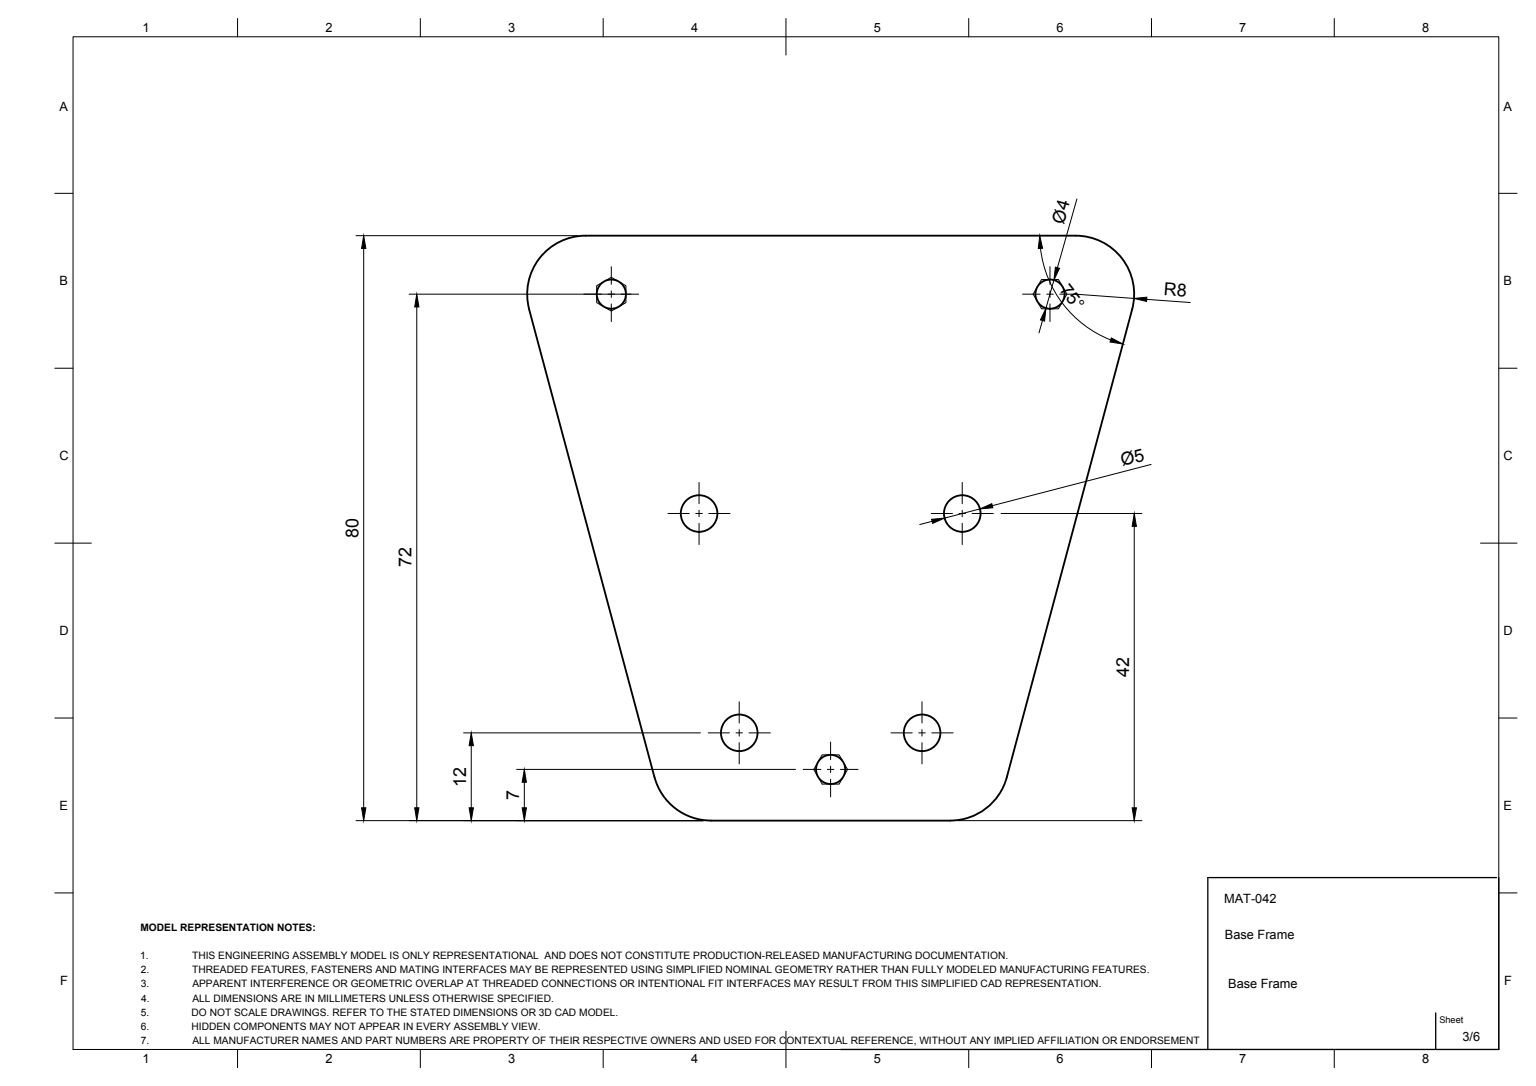
ISO-10303-21;
HEADER;
/* Generated by software containing ST-Developer
 * from STEP Tools, Inc. (www.steptools.com) 
 */

FILE_DESCRIPTION(
/* description */ ('STEP AP214'),
/* implementation_level */ '2;1');

FILE_NAME(
/* name */ 'Base Frame.step',
/* time_stamp */ '2026-11-14T22:03:06-08:00',
/* author */ (''),
/* organization */ (''),
/* preprocessor_version */ 'ST-DEVELOPER v20.2',
/* originating_system */ 'Autodesk Translation Framework v15.17.0.0',
/* authorisation */ '');

FILE_SCHEMA (('AUTOMOTIVE_DESIGN { 1 0 10303 214 3 1 1 }'));
ENDSEC;

DATA;
#10=MECHANICAL_DESIGN_GEOMETRIC_PRESENTATION_REPRESENTATION('',(#303,#304,#305,#306,#307),#12966);
#287=SHAPE_REPRESENTATION_RELATIONSHIP('SRR','None',#13025,#295);
#295=ADVANCED_BREP_SHAPE_REPRESENTATION('',(#315,#316,#317,#318,#319),#12958);
#303=STYLED_ITEM('',(#13074),#315);
#304=STYLED_ITEM('',(#13074),#316);
#305=STYLED_ITEM('',(#13074),#317);
#306=STYLED_ITEM('',(#13074),#318);
#307=STYLED_ITEM('',(#13074),#319);
#315=MANIFOLD_SOLID_BREP('Body1',#5578);
#316=MANIFOLD_SOLID_BREP('Body2',#5579);
#317=MANIFOLD_SOLID_BREP('Body3',#5580);
#318=MANIFOLD_SOLID_BREP('Body4',#5581);
#319=MANIFOLD_SOLID_BREP('Body5',#5582);
#327=FACE_BOUND('',#877,.T.);
#328=FACE_BOUND('',#878,.T.);
#329=FACE_BOUND('',#879,.T.);
#330=FACE_BOUND('',#880,.T.);
#331=FACE_BOUND('',#881,.T.);
#332=FACE_BOUND('',#882,.T.);
#333=FACE_BOUND('',#883,.T.);
#334=FACE_BOUND('',#885,.T.);
#335=FACE_BOUND('',#886,.T.);
#336=FACE_BOUND('',#887,.T.);
#337=FACE_BOUND('',#888,.T.);
#338=FACE_BOUND('',#889,.T.);
#339=FACE_BOUND('',#890,.T.);
#340=FACE_BOUND('',#891,.T.);
#341=FACE_BOUND('',#908,.T.);
#342=FACE_BOUND('',#909,.T.);
#343=FACE_BOUND('',#910,.T.);
#344=FACE_BOUND('',#911,.T.);
#345=FACE_BOUND('',#912,.T.);
#346=FACE_BOUND('',#913,.T.);
#347=FACE_BOUND('',#914,.T.);
#348=FACE_BOUND('',#916,.T.);
#349=FACE_BOUND('',#917,.T.);
#350=FACE_BOUND('',#918,.T.);
#351=FACE_BOUND('',#919,.T.);
#352=FACE_BOUND('',#920,.T.);
#353=FACE_BOUND('',#921,.T.);
#354=FACE_BOUND('',#922,.T.);
#389=PLANE('',#5705);
#390=PLANE('',#5709);
#391=PLANE('',#5713);
#392=PLANE('',#5717);
#393=PLANE('',#5718);
#394=PLANE('',#5719);
#395=PLANE('',#5744);
#396=PLANE('',#5748);
#397=PLANE('',#5752);
#398=PLANE('',#5756);
#399=PLANE('',#5757);
#400=PLANE('',#5758);
#401=PLANE('',#5759);
#402=PLANE('',#5760);
#403=PLANE('',#5761);
#404=PLANE('',#5762);
#405=PLANE('',#5763);
#406=PLANE('',#5764);
#407=PLANE('',#5765);
#408=PLANE('',#5766);
#409=PLANE('',#5767);
#410=PLANE('',#5768);
#411=PLANE('',#5769);
#412=PLANE('',#5770);
#413=PLANE('',#5771);
#414=PLANE('',#5772);
#415=PLANE('',#5773);
#416=PLANE('',#5774);
#417=PLANE('',#5775);
#418=PLANE('',#5776);
#419=PLANE('',#5777);
#420=PLANE('',#5778);
#421=PLANE('',#5779);
#422=PLANE('',#5780);
#423=PLANE('',#5781);
#424=PLANE('',#5782);
#550=FACE_OUTER_BOUND('',#861,.T.);
#551=FACE_OUTER_BOUND('',#862,.T.);
#552=FACE_OUTER_BOUND('',#863,.T.);
#553=FACE_OUTER_BOUND('',#864,.T.);
#554=FACE_OUTER_BOUND('',#865,.T.);
#555=FACE_OUTER_BOUND('',#866,.T.);
#556=FACE_OUTER_BOUND('',#867,.T.);
#557=FACE_OUTER_BOUND('',#868,.T.);
#558=FACE_OUTER_BOUND('',#869,.T.);
#559=FACE_OUTER_BOUND('',#870,.T.);
#560=FACE_OUTER_BOUND('',#871,.T.);
#561=FACE_OUTER_BOUND('',#872,.T.);
#562=FACE_OUTER_BOUND('',#873,.T.);
#563=FACE_OUTER_BOUND('',#874,.T.);
#564=FACE_OUTER_BOUND('',#875,.T.);
#565=FACE_OUTER_BOUND('',#876,.T.);
#566=FACE_OUTER_BOUND('',#884,.T.);
#567=FACE_OUTER_BOUND('',#892,.T.);
#568=FACE_OUTER_BOUND('',#893,.T.);
#569=FACE_OUTER_BOUND('',#894,.T.);
#570=FACE_OUTER_BOUND('',#895,.T.);
#571=FACE_OUTER_BOUND('',#896,.T.);
#572=FACE_OUTER_BOUND('',#897,.T.);
#573=FACE_OUTER_BOUND('',#898,.T.);
#574=FACE_OUTER_BOUND('',#899,.T.);
#575=FACE_OUTER_BOUND('',#900,.T.);
#576=FACE_OUTER_BOUND('',#901,.T.);
#577=FACE_OUTER_BOUND('',#902,.T.);
#578=FACE_OUTER_BOUND('',#903,.T.);
#579=FACE_OUTER_BOUND('',#904,.T.);
#580=FACE_OUTER_BOUND('',#905,.T.);
#581=FACE_OUTER_BOUND('',#906,.T.);
#582=FACE_OUTER_BOUND('',#907,.T.);
#583=FACE_OUTER_BOUND('',#915,.T.);
#584=FACE_OUTER_BOUND('',#923,.T.);
#585=FACE_OUTER_BOUND('',#924,.T.);
#586=FACE_OUTER_BOUND('',#925,.T.);
#587=FACE_OUTER_BOUND('',#926,.T.);
#588=FACE_OUTER_BOUND('',#927,.T.);
#589=FACE_OUTER_BOUND('',#928,.T.);
#590=FACE_OUTER_BOUND('',#929,.T.);
#591=FACE_OUTER_BOUND('',#930,.T.);
#592=FACE_OUTER_BOUND('',#931,.T.);
#593=FACE_OUTER_BOUND('',#932,.T.);
#594=FACE_OUTER_BOUND('',#933,.T.);
#595=FACE_OUTER_BOUND('',#934,.T.);
#596=FACE_OUTER_BOUND('',#935,.T.);
#597=FACE_OUTER_BOUND('',#936,.T.);
#598=FACE_OUTER_BOUND('',#937,.T.);
#599=FACE_OUTER_BOUND('',#938,.T.);
#600=FACE_OUTER_BOUND('',#939,.T.);
#601=FACE_OUTER_BOUND('',#940,.T.);
#602=FACE_OUTER_BOUND('',#941,.T.);
#603=FACE_OUTER_BOUND('',#942,.T.);
#604=FACE_OUTER_BOUND('',#943,.T.);
#605=FACE_OUTER_BOUND('',#944,.T.);
#606=FACE_OUTER_BOUND('',#945,.T.);
#607=FACE_OUTER_BOUND('',#946,.T.);
#861=EDGE_LOOP('',(#3643,#3644,#3645,#3646));
#862=EDGE_LOOP('',(#3647,#3648,#3649,#3650));
#863=EDGE_LOOP('',(#3651,#3652,#3653,#3654));
#864=EDGE_LOOP('',(#3655,#3656,#3657,#3658));
#865=EDGE_LOOP('',(#3659,#3660,#3661,#3662));
#866=EDGE_LOOP('',(#3663,#3664,#3665,#3666));
#867=EDGE_LOOP('',(#3667,#3668,#3669,#3670));
#868=EDGE_LOOP('',(#3671,#3672,#3673,#3674));
#869=EDGE_LOOP('',(#3675,#3676,#3677,#3678));
#870=EDGE_LOOP('',(#3679,#3680,#3681,#3682));
#871=EDGE_LOOP('',(#3683,#3684,#3685,#3686));
#872=EDGE_LOOP('',(#3687,#3688,#3689,#3690));
#873=EDGE_LOOP('',(#3691,#3692,#3693,#3694));
#874=EDGE_LOOP('',(#3695,#3696,#3697,#3698));
#875=EDGE_LOOP('',(#3699,#3700,#3701,#3702));
#876=EDGE_LOOP('',(#3703,#3704,#3705,#3706,#3707,#3708,#3709,#3710));
#877=EDGE_LOOP('',(#3711));
#878=EDGE_LOOP('',(#3712));
#879=EDGE_LOOP('',(#3713));
#880=EDGE_LOOP('',(#3714));
#881=EDGE_LOOP('',(#3715));
#882=EDGE_LOOP('',(#3716));
#883=EDGE_LOOP('',(#3717));
#884=EDGE_LOOP('',(#3718,#3719,#3720,#3721,#3722,#3723,#3724,#3725));
#885=EDGE_LOOP('',(#3726));
#886=EDGE_LOOP('',(#3727));
#887=EDGE_LOOP('',(#3728));
#888=EDGE_LOOP('',(#3729));
#889=EDGE_LOOP('',(#3730));
#890=EDGE_LOOP('',(#3731));
#891=EDGE_LOOP('',(#3732));
#892=EDGE_LOOP('',(#3733,#3734,#3735,#3736));
#893=EDGE_LOOP('',(#3737,#3738,#3739,#3740));
#894=EDGE_LOOP('',(#3741,#3742,#3743,#3744));
#895=EDGE_LOOP('',(#3745,#3746,#3747,#3748));
#896=EDGE_LOOP('',(#3749,#3750,#3751,#3752));
#897=EDGE_LOOP('',(#3753,#3754,#3755,#3756));
#898=EDGE_LOOP('',(#3757,#3758,#3759,#3760));
#899=EDGE_LOOP('',(#3761,#3762,#3763,#3764));
#900=EDGE_LOOP('',(#3765,#3766,#3767,#3768));
#901=EDGE_LOOP('',(#3769,#3770,#3771,#3772));
#902=EDGE_LOOP('',(#3773,#3774,#3775,#3776));
#903=EDGE_LOOP('',(#3777,#3778,#3779,#3780));
#904=EDGE_LOOP('',(#3781,#3782,#3783,#3784));
#905=EDGE_LOOP('',(#3785,#3786,#3787,#3788));
#906=EDGE_LOOP('',(#3789,#3790,#3791,#3792));
#907=EDGE_LOOP('',(#3793,#3794,#3795,#3796,#3797,#3798,#3799,#3800));
#908=EDGE_LOOP('',(#3801));
#909=EDGE_LOOP('',(#3802));
#910=EDGE_LOOP('',(#3803));
#911=EDGE_LOOP('',(#3804));
#912=EDGE_LOOP('',(#3805));
#913=EDGE_LOOP('',(#3806));
#914=EDGE_LOOP('',(#3807));
#915=EDGE_LOOP('',(#3808,#3809,#3810,#3811,#3812,#3813,#3814,#3815));
#916=EDGE_LOOP('',(#3816));
#917=EDGE_LOOP('',(#3817));
#918=EDGE_LOOP('',(#3818));
#919=EDGE_LOOP('',(#3819));
#920=EDGE_LOOP('',(#3820));
#921=EDGE_LOOP('',(#3821));
#922=EDGE_LOOP('',(#3822));
#923=EDGE_LOOP('',(#3823,#3824,#3825,#3826));
#924=EDGE_LOOP('',(#3827,#3828,#3829,#3830));
#925=EDGE_LOOP('',(#3831,#3832,#3833,#3834));
#926=EDGE_LOOP('',(#3835,#3836,#3837,#3838));
#927=EDGE_LOOP('',(#3839,#3840,#3841,#3842));
#928=EDGE_LOOP('',(#3843,#3844,#3845,#3846));
#929=EDGE_LOOP('',(#3847,#3848,#3849,#3850,#3851,#3852));
#930=EDGE_LOOP('',(#3853,#3854,#3855,#3856,#3857,#3858));
#931=EDGE_LOOP('',(#3859,#3860,#3861,#3862));
#932=EDGE_LOOP('',(#3863,#3864,#3865,#3866));
#933=EDGE_LOOP('',(#3867,#3868,#3869,#3870));
#934=EDGE_LOOP('',(#3871,#3872,#3873,#3874));
#935=EDGE_LOOP('',(#3875,#3876,#3877,#3878));
#936=EDGE_LOOP('',(#3879,#3880,#3881,#3882));
#937=EDGE_LOOP('',(#3883,#3884,#3885,#3886,#3887,#3888));
#938=EDGE_LOOP('',(#3889,#3890,#3891,#3892,#3893,#3894));
#939=EDGE_LOOP('',(#3895,#3896,#3897,#3898));
#940=EDGE_LOOP('',(#3899,#3900,#3901,#3902));
#941=EDGE_LOOP('',(#3903,#3904,#3905,#3906));
#942=EDGE_LOOP('',(#3907,#3908,#3909,#3910));
#943=EDGE_LOOP('',(#3911,#3912,#3913,#3914));
#944=EDGE_LOOP('',(#3915,#3916,#3917,#3918));
#945=EDGE_LOOP('',(#3919,#3920,#3921,#3922,#3923,#3924));
#946=EDGE_LOOP('',(#3925,#3926,#3927,#3928,#3929,#3930));
#1234=LINE('',#7771,#1691);
#1235=LINE('',#7777,#1692);
#1236=LINE('',#7783,#1693);
#1237=LINE('',#7789,#1694);
#1238=LINE('',#7795,#1695);
#1239=LINE('',#7801,#1696);
#1240=LINE('',#7807,#1697);
#1241=LINE('',#7814,#1698);
#1242=LINE('',#7817,#1699);
#1243=LINE('',#7820,#1700);
#1244=LINE('',#7822,#1701);
#1245=LINE('',#7823,#1702);
#1246=LINE('',#7828,#1703);
#1247=LINE('',#7832,#1704);
#1248=LINE('',#7834,#1705);
#1249=LINE('',#7835,#1706);
#1250=LINE('',#7840,#1707);
#1251=LINE('',#7844,#1708);
#1252=LINE('',#7846,#1709);
#1253=LINE('',#7847,#1710);
#1254=LINE('',#7852,#1711);
#1255=LINE('',#7855,#1712);
#1256=LINE('',#7856,#1713);
#1257=LINE('',#7863,#1714);
#1258=LINE('',#7869,#1715);
#1259=LINE('',#7875,#1716);
#1260=LINE('',#7881,#1717);
#1261=LINE('',#7888,#1718);
#1262=LINE('',#7891,#1719);
#1263=LINE('',#7896,#1720);
#1264=LINE('',#7902,#1721);
#1265=LINE('',#7908,#1722);
#1266=LINE('',#7912,#1723);
#1267=LINE('',#7914,#1724);
#1268=LINE('',#7915,#1725);
#1269=LINE('',#7920,#1726);
#1270=LINE('',#7924,#1727);
#1271=LINE('',#7926,#1728);
#1272=LINE('',#7927,#1729);
#1273=LINE('',#7932,#1730);
#1274=LINE('',#7936,#1731);
#1275=LINE('',#7938,#1732);
#1276=LINE('',#7939,#1733);
#1277=LINE('',#7944,#1734);
#1278=LINE('',#7947,#1735);
#1279=LINE('',#7948,#1736);
#1280=LINE('',#7954,#1737);
#1281=LINE('',#7956,#1738);
#1282=LINE('',#7958,#1739);
#1283=LINE('',#7959,#1740);
#1284=LINE('',#7962,#1741);
#1285=LINE('',#7964,#1742);
#1286=LINE('',#7965,#1743);
#1287=LINE('',#7968,#1744);
#1288=LINE('',#7970,#1745);
#1289=LINE('',#7971,#1746);
#1290=LINE('',#7974,#1747);
#1291=LINE('',#7976,#1748);
#1292=LINE('',#7977,#1749);
#1293=LINE('',#7980,#1750);
#1294=LINE('',#7982,#1751);
#1295=LINE('',#7983,#1752);
#1296=LINE('',#7985,#1753);
#1297=LINE('',#7986,#1754);
#1298=LINE('',#7992,#1755);
#1299=LINE('',#7994,#1756);
#1300=LINE('',#7996,#1757);
#1301=LINE('',#7997,#1758);
#1302=LINE('',#8000,#1759);
#1303=LINE('',#8002,#1760);
#1304=LINE('',#8003,#1761);
#1305=LINE('',#8006,#1762);
#1306=LINE('',#8008,#1763);
#1307=LINE('',#8009,#1764);
#1308=LINE('',#8012,#1765);
#1309=LINE('',#8014,#1766);
#1310=LINE('',#8015,#1767);
#1311=LINE('',#8018,#1768);
#1312=LINE('',#8020,#1769);
#1313=LINE('',#8021,#1770);
#1314=LINE('',#8023,#1771);
#1315=LINE('',#8024,#1772);
#1316=LINE('',#8030,#1773);
#1317=LINE('',#8032,#1774);
#1318=LINE('',#8034,#1775);
#1319=LINE('',#8035,#1776);
#1320=LINE('',#8038,#1777);
#1321=LINE('',#8040,#1778);
#1322=LINE('',#8041,#1779);
#1323=LINE('',#8044,#1780);
#1324=LINE('',#8046,#1781);
#1325=LINE('',#8047,#1782);
#1326=LINE('',#8050,#1783);
#1327=LINE('',#8052,#1784);
#1328=LINE('',#8053,#1785);
#1329=LINE('',#8056,#1786);
#1330=LINE('',#8058,#1787);
#1331=LINE('',#8059,#1788);
#1332=LINE('',#8061,#1789);
#1333=LINE('',#8062,#1790);
#1691=VECTOR('',#6230,1.99999999999998);
#1692=VECTOR('',#6237,1.99999999999998);
#1693=VECTOR('',#6244,2.);
#1694=VECTOR('',#6251,2.5);
#1695=VECTOR('',#6258,2.5);
#1696=VECTOR('',#6265,2.5);
#1697=VECTOR('',#6272,2.5);
#1698=VECTOR('',#6279,1000.);
#1699=VECTOR('',#6282,1000.);
#1700=VECTOR('',#6285,1000.);
#1701=VECTOR('',#6286,1000.);
#1702=VECTOR('',#6287,1000.);
#1703=VECTOR('',#6292,1000.);
#1704=VECTOR('',#6297,1000.);
#1705=VECTOR('',#6298,1000.);
#1706=VECTOR('',#6299,1000.);
#1707=VECTOR('',#6304,1000.);
#1708=VECTOR('',#6309,1000.);
#1709=VECTOR('',#6310,1000.);
#1710=VECTOR('',#6311,1000.);
#1711=VECTOR('',#6316,1000.);
#1712=VECTOR('',#6321,1000.);
#1713=VECTOR('',#6322,1000.);
#1714=VECTOR('',#6331,1.99999999999998);
#1715=VECTOR('',#6338,1.99999999999998);
#1716=VECTOR('',#6345,2.5);
#1717=VECTOR('',#6352,2.5);
#1718=VECTOR('',#6359,1000.);
#1719=VECTOR('',#6362,1000.);
#1720=VECTOR('',#6367,2.5);
#1721=VECTOR('',#6374,2.5);
#1722=VECTOR('',#6381,2.);
#1723=VECTOR('',#6386,1000.);
#1724=VECTOR('',#6387,1000.);
#1725=VECTOR('',#6388,1000.);
#1726=VECTOR('',#6393,1000.);
#1727=VECTOR('',#6398,1000.);
#1728=VECTOR('',#6399,1000.);
#1729=VECTOR('',#6400,1000.);
#1730=VECTOR('',#6405,1000.);
#1731=VECTOR('',#6410,1000.);
#1732=VECTOR('',#6411,1000.);
#1733=VECTOR('',#6412,1000.);
#1734=VECTOR('',#6417,1000.);
#1735=VECTOR('',#6422,1000.);
#1736=VECTOR('',#6423,1000.);
#1737=VECTOR('',#6430,1000.);
#1738=VECTOR('',#6431,1000.);
#1739=VECTOR('',#6432,1000.);
#1740=VECTOR('',#6433,1000.);
#1741=VECTOR('',#6436,1000.);
#1742=VECTOR('',#6437,1000.);
#1743=VECTOR('',#6438,1000.);
#1744=VECTOR('',#6441,1000.);
#1745=VECTOR('',#6442,1000.);
#1746=VECTOR('',#6443,1000.);
#1747=VECTOR('',#6446,1000.);
#1748=VECTOR('',#6447,1000.);
#1749=VECTOR('',#6448,1000.);
#1750=VECTOR('',#6451,1000.);
#1751=VECTOR('',#6452,1000.);
#1752=VECTOR('',#6453,1000.);
#1753=VECTOR('',#6456,1000.);
#1754=VECTOR('',#6457,1000.);
#1755=VECTOR('',#6464,1000.);
#1756=VECTOR('',#6465,1000.);
#1757=VECTOR('',#6466,1000.);
#1758=VECTOR('',#6467,1000.);
#1759=VECTOR('',#6470,1000.);
#1760=VECTOR('',#6471,1000.);
#1761=VECTOR('',#6472,1000.);
#1762=VECTOR('',#6475,1000.);
#1763=VECTOR('',#6476,1000.);
#1764=VECTOR('',#6477,1000.);
#1765=VECTOR('',#6480,1000.);
#1766=VECTOR('',#6481,1000.);
#1767=VECTOR('',#6482,1000.);
#1768=VECTOR('',#6485,1000.);
#1769=VECTOR('',#6486,1000.);
#1770=VECTOR('',#6487,1000.);
#1771=VECTOR('',#6490,1000.);
#1772=VECTOR('',#6491,1000.);
#1773=VECTOR('',#6498,1000.);
#1774=VECTOR('',#6499,1000.);
#1775=VECTOR('',#6500,1000.);
#1776=VECTOR('',#6501,1000.);
#1777=VECTOR('',#6504,1000.);
#1778=VECTOR('',#6505,1000.);
#1779=VECTOR('',#6506,1000.);
#1780=VECTOR('',#6509,1000.);
#1781=VECTOR('',#6510,1000.);
#1782=VECTOR('',#6511,1000.);
#1783=VECTOR('',#6514,1000.);
#1784=VECTOR('',#6515,1000.);
#1785=VECTOR('',#6516,1000.);
#1786=VECTOR('',#6519,1000.);
#1787=VECTOR('',#6520,1000.);
#1788=VECTOR('',#6521,1000.);
#1789=VECTOR('',#6524,1000.);
#1790=VECTOR('',#6525,1000.);
#2148=CIRCLE('',#5682,1.99999999999998);
#2149=CIRCLE('',#5683,1.99999999999997);
#2150=CIRCLE('',#5685,1.99999999999998);
#2151=CIRCLE('',#5686,1.99999999999997);
#2152=CIRCLE('',#5688,2.);
#2153=CIRCLE('',#5689,2.);
#2154=CIRCLE('',#5691,2.5);
#2155=CIRCLE('',#5692,2.5);
#2156=CIRCLE('',#5694,2.5);
#2157=CIRCLE('',#5695,2.5);
#2158=CIRCLE('',#5697,2.5);
#2159=CIRCLE('',#5698,2.5);
#2160=CIRCLE('',#5700,2.5);
#2161=CIRCLE('',#5701,2.5);
#2162=CIRCLE('',#5703,8.);
#2163=CIRCLE('',#5704,8.00000000000001);
#2164=CIRCLE('',#5707,8.);
#2165=CIRCLE('',#5708,8.);
#2166=CIRCLE('',#5711,8.);
#2167=CIRCLE('',#5712,8.);
#2168=CIRCLE('',#5715,8.00000000000001);
#2169=CIRCLE('',#5716,8.00000000000001);
#2170=CIRCLE('',#5721,1.99999999999998);
#2171=CIRCLE('',#5722,1.99999999999998);
#2172=CIRCLE('',#5724,1.99999999999998);
#2173=CIRCLE('',#5725,1.99999999999998);
#2174=CIRCLE('',#5727,2.5);
#2175=CIRCLE('',#5728,2.5);
#2176=CIRCLE('',#5730,2.5);
#2177=CIRCLE('',#5731,2.5);
#2178=CIRCLE('',#5733,8.00000000000001);
#2179=CIRCLE('',#5734,8.);
#2180=CIRCLE('',#5736,2.5);
#2181=CIRCLE('',#5737,2.5);
#2182=CIRCLE('',#5739,2.5);
#2183=CIRCLE('',#5740,2.5);
#2184=CIRCLE('',#5742,2.);
#2185=CIRCLE('',#5743,2.);
#2186=CIRCLE('',#5746,8.);
#2187=CIRCLE('',#5747,8.00000000000001);
#2188=CIRCLE('',#5750,8.);
#2189=CIRCLE('',#5751,8.);
#2190=CIRCLE('',#5754,8.);
#2191=CIRCLE('',#5755,8.);
#2376=VERTEX_POINT('',#7768);
#2377=VERTEX_POINT('',#7770);
#2378=VERTEX_POINT('',#7774);
#2379=VERTEX_POINT('',#7776);
#2380=VERTEX_POINT('',#7780);
#2381=VERTEX_POINT('',#7782);
#2382=VERTEX_POINT('',#7786);
#2383=VERTEX_POINT('',#7788);
#2384=VERTEX_POINT('',#7792);
#2385=VERTEX_POINT('',#7794);
#2386=VERTEX_POINT('',#7798);
#2387=VERTEX_POINT('',#7800);
#2388=VERTEX_POINT('',#7804);
#2389=VERTEX_POINT('',#7806);
#2390=VERTEX_POINT('',#7810);
#2391=VERTEX_POINT('',#7811);
#2392=VERTEX_POINT('',#7813);
#2393=VERTEX_POINT('',#7815);
#2394=VERTEX_POINT('',#7819);
#2395=VERTEX_POINT('',#7821);
#2396=VERTEX_POINT('',#7825);
#2397=VERTEX_POINT('',#7827);
#2398=VERTEX_POINT('',#7831);
#2399=VERTEX_POINT('',#7833);
#2400=VERTEX_POINT('',#7837);
#2401=VERTEX_POINT('',#7839);
#2402=VERTEX_POINT('',#7843);
#2403=VERTEX_POINT('',#7845);
#2404=VERTEX_POINT('',#7849);
#2405=VERTEX_POINT('',#7851);
#2406=VERTEX_POINT('',#7860);
#2407=VERTEX_POINT('',#7862);
#2408=VERTEX_POINT('',#7866);
#2409=VERTEX_POINT('',#7868);
#2410=VERTEX_POINT('',#7872);
#2411=VERTEX_POINT('',#7874);
#2412=VERTEX_POINT('',#7878);
#2413=VERTEX_POINT('',#7880);
#2414=VERTEX_POINT('',#7884);
#2415=VERTEX_POINT('',#7885);
#2416=VERTEX_POINT('',#7887);
#2417=VERTEX_POINT('',#7889);
#2418=VERTEX_POINT('',#7893);
#2419=VERTEX_POINT('',#7895);
#2420=VERTEX_POINT('',#7899);
#2421=VERTEX_POINT('',#7901);
#2422=VERTEX_POINT('',#7905);
#2423=VERTEX_POINT('',#7907);
#2424=VERTEX_POINT('',#7911);
#2425=VERTEX_POINT('',#7913);
#2426=VERTEX_POINT('',#7917);
#2427=VERTEX_POINT('',#7919);
#2428=VERTEX_POINT('',#7923);
#2429=VERTEX_POINT('',#7925);
#2430=VERTEX_POINT('',#7929);
#2431=VERTEX_POINT('',#7931);
#2432=VERTEX_POINT('',#7935);
#2433=VERTEX_POINT('',#7937);
#2434=VERTEX_POINT('',#7941);
#2435=VERTEX_POINT('',#7943);
#2436=VERTEX_POINT('',#7952);
#2437=VERTEX_POINT('',#7953);
#2438=VERTEX_POINT('',#7955);
#2439=VERTEX_POINT('',#7957);
#2440=VERTEX_POINT('',#7961);
#2441=VERTEX_POINT('',#7963);
#2442=VERTEX_POINT('',#7967);
#2443=VERTEX_POINT('',#7969);
#2444=VERTEX_POINT('',#7973);
#2445=VERTEX_POINT('',#7975);
#2446=VERTEX_POINT('',#7979);
#2447=VERTEX_POINT('',#7981);
#2448=VERTEX_POINT('',#7990);
#2449=VERTEX_POINT('',#7991);
#2450=VERTEX_POINT('',#7993);
#2451=VERTEX_POINT('',#7995);
#2452=VERTEX_POINT('',#7999);
#2453=VERTEX_POINT('',#8001);
#2454=VERTEX_POINT('',#8005);
#2455=VERTEX_POINT('',#8007);
#2456=VERTEX_POINT('',#8011);
#2457=VERTEX_POINT('',#8013);
#2458=VERTEX_POINT('',#8017);
#2459=VERTEX_POINT('',#8019);
#2460=VERTEX_POINT('',#8028);
#2461=VERTEX_POINT('',#8029);
#2462=VERTEX_POINT('',#8031);
#2463=VERTEX_POINT('',#8033);
#2464=VERTEX_POINT('',#8037);
#2465=VERTEX_POINT('',#8039);
#2466=VERTEX_POINT('',#8043);
#2467=VERTEX_POINT('',#8045);
#2468=VERTEX_POINT('',#8049);
#2469=VERTEX_POINT('',#8051);
#2470=VERTEX_POINT('',#8055);
#2471=VERTEX_POINT('',#8057);
#2878=EDGE_CURVE('',#2376,#2376,#2148,.T.);
#2879=EDGE_CURVE('',#2376,#2377,#1234,.T.);
#2880=EDGE_CURVE('',#2377,#2377,#2149,.T.);
#2881=EDGE_CURVE('',#2378,#2378,#2150,.T.);
#2882=EDGE_CURVE('',#2378,#2379,#1235,.T.);
#2883=EDGE_CURVE('',#2379,#2379,#2151,.T.);
#2884=EDGE_CURVE('',#2380,#2380,#2152,.T.);
#2885=EDGE_CURVE('',#2380,#2381,#1236,.T.);
#2886=EDGE_CURVE('',#2381,#2381,#2153,.T.);
#2887=EDGE_CURVE('',#2382,#2382,#2154,.T.);
#2888=EDGE_CURVE('',#2382,#2383,#1237,.T.);
#2889=EDGE_CURVE('',#2383,#2383,#2155,.T.);
#2890=EDGE_CURVE('',#2384,#2384,#2156,.T.);
#2891=EDGE_CURVE('',#2384,#2385,#1238,.T.);
#2892=EDGE_CURVE('',#2385,#2385,#2157,.T.);
#2893=EDGE_CURVE('',#2386,#2386,#2158,.T.);
#2894=EDGE_CURVE('',#2386,#2387,#1239,.T.);
#2895=EDGE_CURVE('',#2387,#2387,#2159,.T.);
#2896=EDGE_CURVE('',#2388,#2388,#2160,.T.);
#2897=EDGE_CURVE('',#2388,#2389,#1240,.T.);
#2898=EDGE_CURVE('',#2389,#2389,#2161,.T.);
#2899=EDGE_CURVE('',#2390,#2391,#2162,.T.);
#2900=EDGE_CURVE('',#2390,#2392,#1241,.T.);
#2901=EDGE_CURVE('',#2392,#2393,#2163,.T.);
#2902=EDGE_CURVE('',#2391,#2393,#1242,.T.);
#2903=EDGE_CURVE('',#2393,#2394,#1243,.T.);
#2904=EDGE_CURVE('',#2395,#2394,#1244,.T.);
#2905=EDGE_CURVE('',#2391,#2395,#1245,.T.);
#2906=EDGE_CURVE('',#2394,#2396,#2164,.T.);
#2907=EDGE_CURVE('',#2397,#2396,#1246,.T.);
#2908=EDGE_CURVE('',#2395,#2397,#2165,.T.);
#2909=EDGE_CURVE('',#2396,#2398,#1247,.T.);
#2910=EDGE_CURVE('',#2399,#2398,#1248,.T.);
#2911=EDGE_CURVE('',#2397,#2399,#1249,.T.);
#2912=EDGE_CURVE('',#2398,#2400,#2166,.T.);
#2913=EDGE_CURVE('',#2401,#2400,#1250,.T.);
#2914=EDGE_CURVE('',#2399,#2401,#2167,.T.);
#2915=EDGE_CURVE('',#2400,#2402,#1251,.T.);
#2916=EDGE_CURVE('',#2403,#2402,#1252,.T.);
#2917=EDGE_CURVE('',#2401,#2403,#1253,.T.);
#2918=EDGE_CURVE('',#2402,#2404,#2168,.T.);
#2919=EDGE_CURVE('',#2405,#2404,#1254,.T.);
#2920=EDGE_CURVE('',#2403,#2405,#2169,.T.);
#2921=EDGE_CURVE('',#2392,#2404,#1255,.T.);
#2922=EDGE_CURVE('',#2405,#2390,#1256,.T.);
#2923=EDGE_CURVE('',#2406,#2406,#2170,.T.);
#2924=EDGE_CURVE('',#2406,#2407,#1257,.T.);
#2925=EDGE_CURVE('',#2407,#2407,#2171,.T.);
#2926=EDGE_CURVE('',#2408,#2408,#2172,.T.);
#2927=EDGE_CURVE('',#2408,#2409,#1258,.T.);
#2928=EDGE_CURVE('',#2409,#2409,#2173,.T.);
#2929=EDGE_CURVE('',#2410,#2410,#2174,.T.);
#2930=EDGE_CURVE('',#2410,#2411,#1259,.T.);
#2931=EDGE_CURVE('',#2411,#2411,#2175,.T.);
#2932=EDGE_CURVE('',#2412,#2412,#2176,.T.);
#2933=EDGE_CURVE('',#2412,#2413,#1260,.T.);
#2934=EDGE_CURVE('',#2413,#2413,#2177,.T.);
#2935=EDGE_CURVE('',#2414,#2415,#2178,.T.);
#2936=EDGE_CURVE('',#2415,#2416,#1261,.T.);
#2937=EDGE_CURVE('',#2416,#2417,#2179,.T.);
#2938=EDGE_CURVE('',#2414,#2417,#1262,.T.);
#2939=EDGE_CURVE('',#2418,#2418,#2180,.T.);
#2940=EDGE_CURVE('',#2418,#2419,#1263,.T.);
#2941=EDGE_CURVE('',#2419,#2419,#2181,.T.);
#2942=EDGE_CURVE('',#2420,#2420,#2182,.T.);
#2943=EDGE_CURVE('',#2420,#2421,#1264,.T.);
#2944=EDGE_CURVE('',#2421,#2421,#2183,.T.);
#2945=EDGE_CURVE('',#2422,#2422,#2184,.T.);
#2946=EDGE_CURVE('',#2422,#2423,#1265,.T.);
#2947=EDGE_CURVE('',#2423,#2423,#2185,.T.);
#2948=EDGE_CURVE('',#2415,#2424,#1266,.T.);
#2949=EDGE_CURVE('',#2424,#2425,#1267,.T.);
#2950=EDGE_CURVE('',#2425,#2416,#1268,.T.);
#2951=EDGE_CURVE('',#2424,#2426,#2186,.T.);
#2952=EDGE_CURVE('',#2426,#2427,#1269,.T.);
#2953=EDGE_CURVE('',#2427,#2425,#2187,.T.);
#2954=EDGE_CURVE('',#2426,#2428,#1270,.T.);
#2955=EDGE_CURVE('',#2428,#2429,#1271,.T.);
#2956=EDGE_CURVE('',#2429,#2427,#1272,.T.);
#2957=EDGE_CURVE('',#2428,#2430,#2188,.T.);
#2958=EDGE_CURVE('',#2430,#2431,#1273,.T.);
#2959=EDGE_CURVE('',#2431,#2429,#2189,.T.);
#2960=EDGE_CURVE('',#2432,#2430,#1274,.T.);
#2961=EDGE_CURVE('',#2432,#2433,#1275,.T.);
#2962=EDGE_CURVE('',#2433,#2431,#1276,.T.);
#2963=EDGE_CURVE('',#2432,#2434,#2190,.T.);
#2964=EDGE_CURVE('',#2434,#2435,#1277,.T.);
#2965=EDGE_CURVE('',#2435,#2433,#2191,.T.);
#2966=EDGE_CURVE('',#2434,#2414,#1278,.T.);
#2967=EDGE_CURVE('',#2417,#2435,#1279,.T.);
#2968=EDGE_CURVE('',#2436,#2437,#1280,.T.);
#2969=EDGE_CURVE('',#2438,#2437,#1281,.T.);
#2970=EDGE_CURVE('',#2439,#2438,#1282,.T.);
#2971=EDGE_CURVE('',#2439,#2436,#1283,.T.);
#2972=EDGE_CURVE('',#2437,#2440,#1284,.T.);
#2973=EDGE_CURVE('',#2441,#2440,#1285,.T.);
#2974=EDGE_CURVE('',#2438,#2441,#1286,.T.);
#2975=EDGE_CURVE('',#2440,#2442,#1287,.T.);
#2976=EDGE_CURVE('',#2443,#2442,#1288,.T.);
#2977=EDGE_CURVE('',#2441,#2443,#1289,.T.);
#2978=EDGE_CURVE('',#2442,#2444,#1290,.T.);
#2979=EDGE_CURVE('',#2445,#2444,#1291,.T.);
#2980=EDGE_CURVE('',#2443,#2445,#1292,.T.);
#2981=EDGE_CURVE('',#2444,#2446,#1293,.T.);
#2982=EDGE_CURVE('',#2447,#2446,#1294,.T.);
#2983=EDGE_CURVE('',#2445,#2447,#1295,.T.);
#2984=EDGE_CURVE('',#2446,#2436,#1296,.T.);
#2985=EDGE_CURVE('',#2447,#2439,#1297,.T.);
#2986=EDGE_CURVE('',#2448,#2449,#1298,.T.);
#2987=EDGE_CURVE('',#2450,#2449,#1299,.T.);
#2988=EDGE_CURVE('',#2451,#2450,#1300,.T.);
#2989=EDGE_CURVE('',#2451,#2448,#1301,.T.);
#2990=EDGE_CURVE('',#2449,#2452,#1302,.T.);
#2991=EDGE_CURVE('',#2453,#2452,#1303,.T.);
#2992=EDGE_CURVE('',#2450,#2453,#1304,.T.);
#2993=EDGE_CURVE('',#2452,#2454,#1305,.T.);
#2994=EDGE_CURVE('',#2455,#2454,#1306,.T.);
#2995=EDGE_CURVE('',#2453,#2455,#1307,.T.);
#2996=EDGE_CURVE('',#2454,#2456,#1308,.T.);
#2997=EDGE_CURVE('',#2457,#2456,#1309,.T.);
#2998=EDGE_CURVE('',#2455,#2457,#1310,.T.);
#2999=EDGE_CURVE('',#2456,#2458,#1311,.T.);
#3000=EDGE_CURVE('',#2459,#2458,#1312,.T.);
#3001=EDGE_CURVE('',#2457,#2459,#1313,.T.);
#3002=EDGE_CURVE('',#2458,#2448,#1314,.T.);
#3003=EDGE_CURVE('',#2459,#2451,#1315,.T.);
#3004=EDGE_CURVE('',#2460,#2461,#1316,.T.);
#3005=EDGE_CURVE('',#2462,#2461,#1317,.T.);
#3006=EDGE_CURVE('',#2463,#2462,#1318,.T.);
#3007=EDGE_CURVE('',#2463,#2460,#1319,.T.);
#3008=EDGE_CURVE('',#2461,#2464,#1320,.T.);
#3009=EDGE_CURVE('',#2465,#2464,#1321,.T.);
#3010=EDGE_CURVE('',#2462,#2465,#1322,.T.);
#3011=EDGE_CURVE('',#2464,#2466,#1323,.T.);
#3012=EDGE_CURVE('',#2467,#2466,#1324,.T.);
#3013=EDGE_CURVE('',#2465,#2467,#1325,.T.);
#3014=EDGE_CURVE('',#2466,#2468,#1326,.T.);
#3015=EDGE_CURVE('',#2469,#2468,#1327,.T.);
#3016=EDGE_CURVE('',#2467,#2469,#1328,.T.);
#3017=EDGE_CURVE('',#2468,#2470,#1329,.T.);
#3018=EDGE_CURVE('',#2471,#2470,#1330,.T.);
#3019=EDGE_CURVE('',#2469,#2471,#1331,.T.);
#3020=EDGE_CURVE('',#2470,#2460,#1332,.T.);
#3021=EDGE_CURVE('',#2471,#2463,#1333,.T.);
#3643=ORIENTED_EDGE('',*,*,#2878,.T.);
#3644=ORIENTED_EDGE('',*,*,#2879,.T.);
#3645=ORIENTED_EDGE('',*,*,#2880,.F.);
#3646=ORIENTED_EDGE('',*,*,#2879,.F.);
#3647=ORIENTED_EDGE('',*,*,#2881,.T.);
#3648=ORIENTED_EDGE('',*,*,#2882,.T.);
#3649=ORIENTED_EDGE('',*,*,#2883,.F.);
#3650=ORIENTED_EDGE('',*,*,#2882,.F.);
#3651=ORIENTED_EDGE('',*,*,#2884,.T.);
#3652=ORIENTED_EDGE('',*,*,#2885,.T.);
#3653=ORIENTED_EDGE('',*,*,#2886,.F.);
#3654=ORIENTED_EDGE('',*,*,#2885,.F.);
#3655=ORIENTED_EDGE('',*,*,#2887,.T.);
#3656=ORIENTED_EDGE('',*,*,#2888,.T.);
#3657=ORIENTED_EDGE('',*,*,#2889,.F.);
#3658=ORIENTED_EDGE('',*,*,#2888,.F.);
#3659=ORIENTED_EDGE('',*,*,#2890,.T.);
#3660=ORIENTED_EDGE('',*,*,#2891,.T.);
#3661=ORIENTED_EDGE('',*,*,#2892,.F.);
#3662=ORIENTED_EDGE('',*,*,#2891,.F.);
#3663=ORIENTED_EDGE('',*,*,#2893,.T.);
#3664=ORIENTED_EDGE('',*,*,#2894,.T.);
#3665=ORIENTED_EDGE('',*,*,#2895,.F.);
#3666=ORIENTED_EDGE('',*,*,#2894,.F.);
#3667=ORIENTED_EDGE('',*,*,#2896,.T.);
#3668=ORIENTED_EDGE('',*,*,#2897,.T.);
#3669=ORIENTED_EDGE('',*,*,#2898,.F.);
#3670=ORIENTED_EDGE('',*,*,#2897,.F.);
#3671=ORIENTED_EDGE('',*,*,#2899,.F.);
#3672=ORIENTED_EDGE('',*,*,#2900,.T.);
#3673=ORIENTED_EDGE('',*,*,#2901,.T.);
#3674=ORIENTED_EDGE('',*,*,#2902,.F.);
#3675=ORIENTED_EDGE('',*,*,#2902,.T.);
#3676=ORIENTED_EDGE('',*,*,#2903,.T.);
#3677=ORIENTED_EDGE('',*,*,#2904,.F.);
#3678=ORIENTED_EDGE('',*,*,#2905,.F.);
#3679=ORIENTED_EDGE('',*,*,#2904,.T.);
#3680=ORIENTED_EDGE('',*,*,#2906,.T.);
#3681=ORIENTED_EDGE('',*,*,#2907,.F.);
#3682=ORIENTED_EDGE('',*,*,#2908,.F.);
#3683=ORIENTED_EDGE('',*,*,#2907,.T.);
#3684=ORIENTED_EDGE('',*,*,#2909,.T.);
#3685=ORIENTED_EDGE('',*,*,#2910,.F.);
#3686=ORIENTED_EDGE('',*,*,#2911,.F.);
#3687=ORIENTED_EDGE('',*,*,#2910,.T.);
#3688=ORIENTED_EDGE('',*,*,#2912,.T.);
#3689=ORIENTED_EDGE('',*,*,#2913,.F.);
#3690=ORIENTED_EDGE('',*,*,#2914,.F.);
#3691=ORIENTED_EDGE('',*,*,#2913,.T.);
#3692=ORIENTED_EDGE('',*,*,#2915,.T.);
#3693=ORIENTED_EDGE('',*,*,#2916,.F.);
#3694=ORIENTED_EDGE('',*,*,#2917,.F.);
#3695=ORIENTED_EDGE('',*,*,#2916,.T.);
#3696=ORIENTED_EDGE('',*,*,#2918,.T.);
#3697=ORIENTED_EDGE('',*,*,#2919,.F.);
#3698=ORIENTED_EDGE('',*,*,#2920,.F.);
#3699=ORIENTED_EDGE('',*,*,#2919,.T.);
#3700=ORIENTED_EDGE('',*,*,#2921,.F.);
#3701=ORIENTED_EDGE('',*,*,#2900,.F.);
#3702=ORIENTED_EDGE('',*,*,#2922,.F.);
#3703=ORIENTED_EDGE('',*,*,#2899,.T.);
#3704=ORIENTED_EDGE('',*,*,#2905,.T.);
#3705=ORIENTED_EDGE('',*,*,#2908,.T.);
#3706=ORIENTED_EDGE('',*,*,#2911,.T.);
#3707=ORIENTED_EDGE('',*,*,#2914,.T.);
#3708=ORIENTED_EDGE('',*,*,#2917,.T.);
#3709=ORIENTED_EDGE('',*,*,#2920,.T.);
#3710=ORIENTED_EDGE('',*,*,#2922,.T.);
#3711=ORIENTED_EDGE('',*,*,#2896,.F.);
#3712=ORIENTED_EDGE('',*,*,#2890,.F.);
#3713=ORIENTED_EDGE('',*,*,#2884,.F.);
#3714=ORIENTED_EDGE('',*,*,#2878,.F.);
#3715=ORIENTED_EDGE('',*,*,#2881,.F.);
#3716=ORIENTED_EDGE('',*,*,#2887,.F.);
#3717=ORIENTED_EDGE('',*,*,#2893,.F.);
#3718=ORIENTED_EDGE('',*,*,#2921,.T.);
#3719=ORIENTED_EDGE('',*,*,#2918,.F.);
#3720=ORIENTED_EDGE('',*,*,#2915,.F.);
#3721=ORIENTED_EDGE('',*,*,#2912,.F.);
#3722=ORIENTED_EDGE('',*,*,#2909,.F.);
#3723=ORIENTED_EDGE('',*,*,#2906,.F.);
#3724=ORIENTED_EDGE('',*,*,#2903,.F.);
#3725=ORIENTED_EDGE('',*,*,#2901,.F.);
#3726=ORIENTED_EDGE('',*,*,#2898,.T.);
#3727=ORIENTED_EDGE('',*,*,#2895,.T.);
#3728=ORIENTED_EDGE('',*,*,#2892,.T.);
#3729=ORIENTED_EDGE('',*,*,#2889,.T.);
#3730=ORIENTED_EDGE('',*,*,#2886,.T.);
#3731=ORIENTED_EDGE('',*,*,#2883,.T.);
#3732=ORIENTED_EDGE('',*,*,#2880,.T.);
#3733=ORIENTED_EDGE('',*,*,#2923,.F.);
#3734=ORIENTED_EDGE('',*,*,#2924,.T.);
#3735=ORIENTED_EDGE('',*,*,#2925,.F.);
#3736=ORIENTED_EDGE('',*,*,#2924,.F.);
#3737=ORIENTED_EDGE('',*,*,#2926,.F.);
#3738=ORIENTED_EDGE('',*,*,#2927,.T.);
#3739=ORIENTED_EDGE('',*,*,#2928,.F.);
#3740=ORIENTED_EDGE('',*,*,#2927,.F.);
#3741=ORIENTED_EDGE('',*,*,#2929,.F.);
#3742=ORIENTED_EDGE('',*,*,#2930,.T.);
#3743=ORIENTED_EDGE('',*,*,#2931,.F.);
#3744=ORIENTED_EDGE('',*,*,#2930,.F.);
#3745=ORIENTED_EDGE('',*,*,#2932,.F.);
#3746=ORIENTED_EDGE('',*,*,#2933,.T.);
#3747=ORIENTED_EDGE('',*,*,#2934,.F.);
#3748=ORIENTED_EDGE('',*,*,#2933,.F.);
#3749=ORIENTED_EDGE('',*,*,#2935,.T.);
#3750=ORIENTED_EDGE('',*,*,#2936,.T.);
#3751=ORIENTED_EDGE('',*,*,#2937,.T.);
#3752=ORIENTED_EDGE('',*,*,#2938,.F.);
#3753=ORIENTED_EDGE('',*,*,#2939,.F.);
#3754=ORIENTED_EDGE('',*,*,#2940,.T.);
#3755=ORIENTED_EDGE('',*,*,#2941,.F.);
#3756=ORIENTED_EDGE('',*,*,#2940,.F.);
#3757=ORIENTED_EDGE('',*,*,#2942,.F.);
#3758=ORIENTED_EDGE('',*,*,#2943,.T.);
#3759=ORIENTED_EDGE('',*,*,#2944,.F.);
#3760=ORIENTED_EDGE('',*,*,#2943,.F.);
#3761=ORIENTED_EDGE('',*,*,#2945,.F.);
#3762=ORIENTED_EDGE('',*,*,#2946,.T.);
#3763=ORIENTED_EDGE('',*,*,#2947,.F.);
#3764=ORIENTED_EDGE('',*,*,#2946,.F.);
#3765=ORIENTED_EDGE('',*,*,#2936,.F.);
#3766=ORIENTED_EDGE('',*,*,#2948,.T.);
#3767=ORIENTED_EDGE('',*,*,#2949,.T.);
#3768=ORIENTED_EDGE('',*,*,#2950,.T.);
#3769=ORIENTED_EDGE('',*,*,#2949,.F.);
#3770=ORIENTED_EDGE('',*,*,#2951,.T.);
#3771=ORIENTED_EDGE('',*,*,#2952,.T.);
#3772=ORIENTED_EDGE('',*,*,#2953,.T.);
#3773=ORIENTED_EDGE('',*,*,#2952,.F.);
#3774=ORIENTED_EDGE('',*,*,#2954,.T.);
#3775=ORIENTED_EDGE('',*,*,#2955,.T.);
#3776=ORIENTED_EDGE('',*,*,#2956,.T.);
#3777=ORIENTED_EDGE('',*,*,#2955,.F.);
#3778=ORIENTED_EDGE('',*,*,#2957,.T.);
#3779=ORIENTED_EDGE('',*,*,#2958,.T.);
#3780=ORIENTED_EDGE('',*,*,#2959,.T.);
#3781=ORIENTED_EDGE('',*,*,#2958,.F.);
#3782=ORIENTED_EDGE('',*,*,#2960,.F.);
#3783=ORIENTED_EDGE('',*,*,#2961,.T.);
#3784=ORIENTED_EDGE('',*,*,#2962,.T.);
#3785=ORIENTED_EDGE('',*,*,#2961,.F.);
#3786=ORIENTED_EDGE('',*,*,#2963,.T.);
#3787=ORIENTED_EDGE('',*,*,#2964,.T.);
#3788=ORIENTED_EDGE('',*,*,#2965,.T.);
#3789=ORIENTED_EDGE('',*,*,#2964,.F.);
#3790=ORIENTED_EDGE('',*,*,#2966,.T.);
#3791=ORIENTED_EDGE('',*,*,#2938,.T.);
#3792=ORIENTED_EDGE('',*,*,#2967,.T.);
#3793=ORIENTED_EDGE('',*,*,#2937,.F.);
#3794=ORIENTED_EDGE('',*,*,#2950,.F.);
#3795=ORIENTED_EDGE('',*,*,#2953,.F.);
#3796=ORIENTED_EDGE('',*,*,#2956,.F.);
#3797=ORIENTED_EDGE('',*,*,#2959,.F.);
#3798=ORIENTED_EDGE('',*,*,#2962,.F.);
#3799=ORIENTED_EDGE('',*,*,#2965,.F.);
#3800=ORIENTED_EDGE('',*,*,#2967,.F.);
#3801=ORIENTED_EDGE('',*,*,#2941,.T.);
#3802=ORIENTED_EDGE('',*,*,#2944,.T.);
#3803=ORIENTED_EDGE('',*,*,#2947,.T.);
#3804=ORIENTED_EDGE('',*,*,#2925,.T.);
#3805=ORIENTED_EDGE('',*,*,#2928,.T.);
#3806=ORIENTED_EDGE('',*,*,#2931,.T.);
#3807=ORIENTED_EDGE('',*,*,#2934,.T.);
#3808=ORIENTED_EDGE('',*,*,#2966,.F.);
#3809=ORIENTED_EDGE('',*,*,#2963,.F.);
#3810=ORIENTED_EDGE('',*,*,#2960,.T.);
#3811=ORIENTED_EDGE('',*,*,#2957,.F.);
#3812=ORIENTED_EDGE('',*,*,#2954,.F.);
#3813=ORIENTED_EDGE('',*,*,#2951,.F.);
#3814=ORIENTED_EDGE('',*,*,#2948,.F.);
#3815=ORIENTED_EDGE('',*,*,#2935,.F.);
#3816=ORIENTED_EDGE('',*,*,#2939,.T.);
#3817=ORIENTED_EDGE('',*,*,#2932,.T.);
#3818=ORIENTED_EDGE('',*,*,#2942,.T.);
#3819=ORIENTED_EDGE('',*,*,#2929,.T.);
#3820=ORIENTED_EDGE('',*,*,#2945,.T.);
#3821=ORIENTED_EDGE('',*,*,#2926,.T.);
#3822=ORIENTED_EDGE('',*,*,#2923,.T.);
#3823=ORIENTED_EDGE('',*,*,#2968,.T.);
#3824=ORIENTED_EDGE('',*,*,#2969,.F.);
#3825=ORIENTED_EDGE('',*,*,#2970,.F.);
#3826=ORIENTED_EDGE('',*,*,#2971,.T.);
#3827=ORIENTED_EDGE('',*,*,#2972,.T.);
#3828=ORIENTED_EDGE('',*,*,#2973,.F.);
#3829=ORIENTED_EDGE('',*,*,#2974,.F.);
#3830=ORIENTED_EDGE('',*,*,#2969,.T.);
#3831=ORIENTED_EDGE('',*,*,#2975,.T.);
#3832=ORIENTED_EDGE('',*,*,#2976,.F.);
#3833=ORIENTED_EDGE('',*,*,#2977,.F.);
#3834=ORIENTED_EDGE('',*,*,#2973,.T.);
#3835=ORIENTED_EDGE('',*,*,#2978,.T.);
#3836=ORIENTED_EDGE('',*,*,#2979,.F.);
#3837=ORIENTED_EDGE('',*,*,#2980,.F.);
#3838=ORIENTED_EDGE('',*,*,#2976,.T.);
#3839=ORIENTED_EDGE('',*,*,#2981,.T.);
#3840=ORIENTED_EDGE('',*,*,#2982,.F.);
#3841=ORIENTED_EDGE('',*,*,#2983,.F.);
#3842=ORIENTED_EDGE('',*,*,#2979,.T.);
#3843=ORIENTED_EDGE('',*,*,#2984,.T.);
#3844=ORIENTED_EDGE('',*,*,#2971,.F.);
#3845=ORIENTED_EDGE('',*,*,#2985,.F.);
#3846=ORIENTED_EDGE('',*,*,#2982,.T.);
#3847=ORIENTED_EDGE('',*,*,#2970,.T.);
#3848=ORIENTED_EDGE('',*,*,#2974,.T.);
#3849=ORIENTED_EDGE('',*,*,#2977,.T.);
#3850=ORIENTED_EDGE('',*,*,#2980,.T.);
#3851=ORIENTED_EDGE('',*,*,#2983,.T.);
#3852=ORIENTED_EDGE('',*,*,#2985,.T.);
#3853=ORIENTED_EDGE('',*,*,#2968,.F.);
#3854=ORIENTED_EDGE('',*,*,#2984,.F.);
#3855=ORIENTED_EDGE('',*,*,#2981,.F.);
#3856=ORIENTED_EDGE('',*,*,#2978,.F.);
#3857=ORIENTED_EDGE('',*,*,#2975,.F.);
#3858=ORIENTED_EDGE('',*,*,#2972,.F.);
#3859=ORIENTED_EDGE('',*,*,#2986,.T.);
#3860=ORIENTED_EDGE('',*,*,#2987,.F.);
#3861=ORIENTED_EDGE('',*,*,#2988,.F.);
#3862=ORIENTED_EDGE('',*,*,#2989,.T.);
#3863=ORIENTED_EDGE('',*,*,#2990,.T.);
#3864=ORIENTED_EDGE('',*,*,#2991,.F.);
#3865=ORIENTED_EDGE('',*,*,#2992,.F.);
#3866=ORIENTED_EDGE('',*,*,#2987,.T.);
#3867=ORIENTED_EDGE('',*,*,#2993,.T.);
#3868=ORIENTED_EDGE('',*,*,#2994,.F.);
#3869=ORIENTED_EDGE('',*,*,#2995,.F.);
#3870=ORIENTED_EDGE('',*,*,#2991,.T.);
#3871=ORIENTED_EDGE('',*,*,#2996,.T.);
#3872=ORIENTED_EDGE('',*,*,#2997,.F.);
#3873=ORIENTED_EDGE('',*,*,#2998,.F.);
#3874=ORIENTED_EDGE('',*,*,#2994,.T.);
#3875=ORIENTED_EDGE('',*,*,#2999,.T.);
#3876=ORIENTED_EDGE('',*,*,#3000,.F.);
#3877=ORIENTED_EDGE('',*,*,#3001,.F.);
#3878=ORIENTED_EDGE('',*,*,#2997,.T.);
#3879=ORIENTED_EDGE('',*,*,#3002,.T.);
#3880=ORIENTED_EDGE('',*,*,#2989,.F.);
#3881=ORIENTED_EDGE('',*,*,#3003,.F.);
#3882=ORIENTED_EDGE('',*,*,#3000,.T.);
#3883=ORIENTED_EDGE('',*,*,#2988,.T.);
#3884=ORIENTED_EDGE('',*,*,#2992,.T.);
#3885=ORIENTED_EDGE('',*,*,#2995,.T.);
#3886=ORIENTED_EDGE('',*,*,#2998,.T.);
#3887=ORIENTED_EDGE('',*,*,#3001,.T.);
#3888=ORIENTED_EDGE('',*,*,#3003,.T.);
#3889=ORIENTED_EDGE('',*,*,#2986,.F.);
#3890=ORIENTED_EDGE('',*,*,#3002,.F.);
#3891=ORIENTED_EDGE('',*,*,#2999,.F.);
#3892=ORIENTED_EDGE('',*,*,#2996,.F.);
#3893=ORIENTED_EDGE('',*,*,#2993,.F.);
#3894=ORIENTED_EDGE('',*,*,#2990,.F.);
#3895=ORIENTED_EDGE('',*,*,#3004,.T.);
#3896=ORIENTED_EDGE('',*,*,#3005,.F.);
#3897=ORIENTED_EDGE('',*,*,#3006,.F.);
#3898=ORIENTED_EDGE('',*,*,#3007,.T.);
#3899=ORIENTED_EDGE('',*,*,#3008,.T.);
#3900=ORIENTED_EDGE('',*,*,#3009,.F.);
#3901=ORIENTED_EDGE('',*,*,#3010,.F.);
#3902=ORIENTED_EDGE('',*,*,#3005,.T.);
#3903=ORIENTED_EDGE('',*,*,#3011,.T.);
#3904=ORIENTED_EDGE('',*,*,#3012,.F.);
#3905=ORIENTED_EDGE('',*,*,#3013,.F.);
#3906=ORIENTED_EDGE('',*,*,#3009,.T.);
#3907=ORIENTED_EDGE('',*,*,#3014,.T.);
#3908=ORIENTED_EDGE('',*,*,#3015,.F.);
#3909=ORIENTED_EDGE('',*,*,#3016,.F.);
#3910=ORIENTED_EDGE('',*,*,#3012,.T.);
#3911=ORIENTED_EDGE('',*,*,#3017,.T.);
#3912=ORIENTED_EDGE('',*,*,#3018,.F.);
#3913=ORIENTED_EDGE('',*,*,#3019,.F.);
#3914=ORIENTED_EDGE('',*,*,#3015,.T.);
#3915=ORIENTED_EDGE('',*,*,#3020,.T.);
#3916=ORIENTED_EDGE('',*,*,#3007,.F.);
#3917=ORIENTED_EDGE('',*,*,#3021,.F.);
#3918=ORIENTED_EDGE('',*,*,#3018,.T.);
#3919=ORIENTED_EDGE('',*,*,#3006,.T.);
#3920=ORIENTED_EDGE('',*,*,#3010,.T.);
#3921=ORIENTED_EDGE('',*,*,#3013,.T.);
#3922=ORIENTED_EDGE('',*,*,#3016,.T.);
#3923=ORIENTED_EDGE('',*,*,#3019,.T.);
#3924=ORIENTED_EDGE('',*,*,#3021,.T.);
#3925=ORIENTED_EDGE('',*,*,#3004,.F.);
#3926=ORIENTED_EDGE('',*,*,#3020,.F.);
#3927=ORIENTED_EDGE('',*,*,#3017,.F.);
#3928=ORIENTED_EDGE('',*,*,#3014,.F.);
#3929=ORIENTED_EDGE('',*,*,#3011,.F.);
#3930=ORIENTED_EDGE('',*,*,#3008,.F.);
#5173=CYLINDRICAL_SURFACE('',#5681,1.99999999999998);
#5174=CYLINDRICAL_SURFACE('',#5684,1.99999999999998);
#5175=CYLINDRICAL_SURFACE('',#5687,2.);
#5176=CYLINDRICAL_SURFACE('',#5690,2.5);
#5177=CYLINDRICAL_SURFACE('',#5693,2.5);
#5178=CYLINDRICAL_SURFACE('',#5696,2.5);
#5179=CYLINDRICAL_SURFACE('',#5699,2.5);
#5180=CYLINDRICAL_SURFACE('',#5702,8.00000000000001);
#5181=CYLINDRICAL_SURFACE('',#5706,8.);
#5182=CYLINDRICAL_SURFACE('',#5710,8.);
#5183=CYLINDRICAL_SURFACE('',#5714,8.);
#5184=CYLINDRICAL_SURFACE('',#5720,1.99999999999998);
#5185=CYLINDRICAL_SURFACE('',#5723,1.99999999999998);
#5186=CYLINDRICAL_SURFACE('',#5726,2.5);
#5187=CYLINDRICAL_SURFACE('',#5729,2.5);
#5188=CYLINDRICAL_SURFACE('',#5732,8.00000000000001);
#5189=CYLINDRICAL_SURFACE('',#5735,2.5);
#5190=CYLINDRICAL_SURFACE('',#5738,2.5);
#5191=CYLINDRICAL_SURFACE('',#5741,2.);
#5192=CYLINDRICAL_SURFACE('',#5745,8.);
#5193=CYLINDRICAL_SURFACE('',#5749,8.);
#5194=CYLINDRICAL_SURFACE('',#5753,8.);
#5267=ADVANCED_FACE('',(#550),#5173,.F.);
#5268=ADVANCED_FACE('',(#551),#5174,.F.);
#5269=ADVANCED_FACE('',(#552),#5175,.F.);
#5270=ADVANCED_FACE('',(#553),#5176,.F.);
#5271=ADVANCED_FACE('',(#554),#5177,.F.);
#5272=ADVANCED_FACE('',(#555),#5178,.F.);
#5273=ADVANCED_FACE('',(#556),#5179,.F.);
#5274=ADVANCED_FACE('',(#557),#5180,.T.);
#5275=ADVANCED_FACE('',(#558),#389,.F.);
#5276=ADVANCED_FACE('',(#559),#5181,.T.);
#5277=ADVANCED_FACE('',(#560),#390,.F.);
#5278=ADVANCED_FACE('',(#561),#5182,.T.);
#5279=ADVANCED_FACE('',(#562),#391,.F.);
#5280=ADVANCED_FACE('',(#563),#5183,.T.);
#5281=ADVANCED_FACE('',(#564),#392,.F.);
#5282=ADVANCED_FACE('',(#565,#327,#328,#329,#330,#331,#332,#333),#393,.T.);
#5283=ADVANCED_FACE('',(#566,#334,#335,#336,#337,#338,#339,#340),#394,.F.);
#5284=ADVANCED_FACE('',(#567),#5184,.F.);
#5285=ADVANCED_FACE('',(#568),#5185,.F.);
#5286=ADVANCED_FACE('',(#569),#5186,.F.);
#5287=ADVANCED_FACE('',(#570),#5187,.F.);
#5288=ADVANCED_FACE('',(#571),#5188,.T.);
#5289=ADVANCED_FACE('',(#572),#5189,.F.);
#5290=ADVANCED_FACE('',(#573),#5190,.F.);
#5291=ADVANCED_FACE('',(#574),#5191,.F.);
#5292=ADVANCED_FACE('',(#575),#395,.F.);
#5293=ADVANCED_FACE('',(#576),#5192,.T.);
#5294=ADVANCED_FACE('',(#577),#396,.F.);
#5295=ADVANCED_FACE('',(#578),#5193,.T.);
#5296=ADVANCED_FACE('',(#579),#397,.F.);
#5297=ADVANCED_FACE('',(#580),#5194,.T.);
#5298=ADVANCED_FACE('',(#581),#398,.F.);
#5299=ADVANCED_FACE('',(#582,#341,#342,#343,#344,#345,#346,#347),#399,.F.);
#5300=ADVANCED_FACE('',(#583,#348,#349,#350,#351,#352,#353,#354),#400,.F.);
#5301=ADVANCED_FACE('',(#584),#401,.F.);
#5302=ADVANCED_FACE('',(#585),#402,.F.);
#5303=ADVANCED_FACE('',(#586),#403,.F.);
#5304=ADVANCED_FACE('',(#587),#404,.F.);
#5305=ADVANCED_FACE('',(#588),#405,.F.);
#5306=ADVANCED_FACE('',(#589),#406,.F.);
#5307=ADVANCED_FACE('',(#590),#407,.T.);
#5308=ADVANCED_FACE('',(#591),#408,.F.);
#5309=ADVANCED_FACE('',(#592),#409,.F.);
#5310=ADVANCED_FACE('',(#593),#410,.F.);
#5311=ADVANCED_FACE('',(#594),#411,.F.);
#5312=ADVANCED_FACE('',(#595),#412,.F.);
#5313=ADVANCED_FACE('',(#596),#413,.F.);
#5314=ADVANCED_FACE('',(#597),#414,.F.);
#5315=ADVANCED_FACE('',(#598),#415,.T.);
#5316=ADVANCED_FACE('',(#599),#416,.F.);
#5317=ADVANCED_FACE('',(#600),#417,.F.);
#5318=ADVANCED_FACE('',(#601),#418,.F.);
#5319=ADVANCED_FACE('',(#602),#419,.F.);
#5320=ADVANCED_FACE('',(#603),#420,.F.);
#5321=ADVANCED_FACE('',(#604),#421,.F.);
#5322=ADVANCED_FACE('',(#605),#422,.F.);
#5323=ADVANCED_FACE('',(#606),#423,.T.);
#5324=ADVANCED_FACE('',(#607),#424,.F.);
#5578=CLOSED_SHELL('',(#5267,#5268,#5269,#5270,#5271,#5272,#5273,#5274,
#5275,#5276,#5277,#5278,#5279,#5280,#5281,#5282,#5283));
#5579=CLOSED_SHELL('',(#5284,#5285,#5286,#5287,#5288,#5289,#5290,#5291,
#5292,#5293,#5294,#5295,#5296,#5297,#5298,#5299,#5300));
#5580=CLOSED_SHELL('',(#5301,#5302,#5303,#5304,#5305,#5306,#5307,#5308));
#5581=CLOSED_SHELL('',(#5309,#5310,#5311,#5312,#5313,#5314,#5315,#5316));
#5582=CLOSED_SHELL('',(#5317,#5318,#5319,#5320,#5321,#5322,#5323,#5324));
#5680=AXIS2_PLACEMENT_3D('',#7766,#6224,#6225);
#5681=AXIS2_PLACEMENT_3D('',#7767,#6226,#6227);
#5682=AXIS2_PLACEMENT_3D('',#7769,#6228,#6229);
#5683=AXIS2_PLACEMENT_3D('',#7772,#6231,#6232);
#5684=AXIS2_PLACEMENT_3D('',#7773,#6233,#6234);
#5685=AXIS2_PLACEMENT_3D('',#7775,#6235,#6236);
#5686=AXIS2_PLACEMENT_3D('',#7778,#6238,#6239);
#5687=AXIS2_PLACEMENT_3D('',#7779,#6240,#6241);
#5688=AXIS2_PLACEMENT_3D('',#7781,#6242,#6243);
#5689=AXIS2_PLACEMENT_3D('',#7784,#6245,#6246);
#5690=AXIS2_PLACEMENT_3D('',#7785,#6247,#6248);
#5691=AXIS2_PLACEMENT_3D('',#7787,#6249,#6250);
#5692=AXIS2_PLACEMENT_3D('',#7790,#6252,#6253);
#5693=AXIS2_PLACEMENT_3D('',#7791,#6254,#6255);
#5694=AXIS2_PLACEMENT_3D('',#7793,#6256,#6257);
#5695=AXIS2_PLACEMENT_3D('',#7796,#6259,#6260);
#5696=AXIS2_PLACEMENT_3D('',#7797,#6261,#6262);
#5697=AXIS2_PLACEMENT_3D('',#7799,#6263,#6264);
#5698=AXIS2_PLACEMENT_3D('',#7802,#6266,#6267);
#5699=AXIS2_PLACEMENT_3D('',#7803,#6268,#6269);
#5700=AXIS2_PLACEMENT_3D('',#7805,#6270,#6271);
#5701=AXIS2_PLACEMENT_3D('',#7808,#6273,#6274);
#5702=AXIS2_PLACEMENT_3D('',#7809,#6275,#6276);
#5703=AXIS2_PLACEMENT_3D('',#7812,#6277,#6278);
#5704=AXIS2_PLACEMENT_3D('',#7816,#6280,#6281);
#5705=AXIS2_PLACEMENT_3D('',#7818,#6283,#6284);
#5706=AXIS2_PLACEMENT_3D('',#7824,#6288,#6289);
#5707=AXIS2_PLACEMENT_3D('',#7826,#6290,#6291);
#5708=AXIS2_PLACEMENT_3D('',#7829,#6293,#6294);
#5709=AXIS2_PLACEMENT_3D('',#7830,#6295,#6296);
#5710=AXIS2_PLACEMENT_3D('',#7836,#6300,#6301);
#5711=AXIS2_PLACEMENT_3D('',#7838,#6302,#6303);
#5712=AXIS2_PLACEMENT_3D('',#7841,#6305,#6306);
#5713=AXIS2_PLACEMENT_3D('',#7842,#6307,#6308);
#5714=AXIS2_PLACEMENT_3D('',#7848,#6312,#6313);
#5715=AXIS2_PLACEMENT_3D('',#7850,#6314,#6315);
#5716=AXIS2_PLACEMENT_3D('',#7853,#6317,#6318);
#5717=AXIS2_PLACEMENT_3D('',#7854,#6319,#6320);
#5718=AXIS2_PLACEMENT_3D('',#7857,#6323,#6324);
#5719=AXIS2_PLACEMENT_3D('',#7858,#6325,#6326);
#5720=AXIS2_PLACEMENT_3D('',#7859,#6327,#6328);
#5721=AXIS2_PLACEMENT_3D('',#7861,#6329,#6330);
#5722=AXIS2_PLACEMENT_3D('',#7864,#6332,#6333);
#5723=AXIS2_PLACEMENT_3D('',#7865,#6334,#6335);
#5724=AXIS2_PLACEMENT_3D('',#7867,#6336,#6337);
#5725=AXIS2_PLACEMENT_3D('',#7870,#6339,#6340);
#5726=AXIS2_PLACEMENT_3D('',#7871,#6341,#6342);
#5727=AXIS2_PLACEMENT_3D('',#7873,#6343,#6344);
#5728=AXIS2_PLACEMENT_3D('',#7876,#6346,#6347);
#5729=AXIS2_PLACEMENT_3D('',#7877,#6348,#6349);
#5730=AXIS2_PLACEMENT_3D('',#7879,#6350,#6351);
#5731=AXIS2_PLACEMENT_3D('',#7882,#6353,#6354);
#5732=AXIS2_PLACEMENT_3D('',#7883,#6355,#6356);
#5733=AXIS2_PLACEMENT_3D('',#7886,#6357,#6358);
#5734=AXIS2_PLACEMENT_3D('',#7890,#6360,#6361);
#5735=AXIS2_PLACEMENT_3D('',#7892,#6363,#6364);
#5736=AXIS2_PLACEMENT_3D('',#7894,#6365,#6366);
#5737=AXIS2_PLACEMENT_3D('',#7897,#6368,#6369);
#5738=AXIS2_PLACEMENT_3D('',#7898,#6370,#6371);
#5739=AXIS2_PLACEMENT_3D('',#7900,#6372,#6373);
#5740=AXIS2_PLACEMENT_3D('',#7903,#6375,#6376);
#5741=AXIS2_PLACEMENT_3D('',#7904,#6377,#6378);
#5742=AXIS2_PLACEMENT_3D('',#7906,#6379,#6380);
#5743=AXIS2_PLACEMENT_3D('',#7909,#6382,#6383);
#5744=AXIS2_PLACEMENT_3D('',#7910,#6384,#6385);
#5745=AXIS2_PLACEMENT_3D('',#7916,#6389,#6390);
#5746=AXIS2_PLACEMENT_3D('',#7918,#6391,#6392);
#5747=AXIS2_PLACEMENT_3D('',#7921,#6394,#6395);
#5748=AXIS2_PLACEMENT_3D('',#7922,#6396,#6397);
#5749=AXIS2_PLACEMENT_3D('',#7928,#6401,#6402);
#5750=AXIS2_PLACEMENT_3D('',#7930,#6403,#6404);
#5751=AXIS2_PLACEMENT_3D('',#7933,#6406,#6407);
#5752=AXIS2_PLACEMENT_3D('',#7934,#6408,#6409);
#5753=AXIS2_PLACEMENT_3D('',#7940,#6413,#6414);
#5754=AXIS2_PLACEMENT_3D('',#7942,#6415,#6416);
#5755=AXIS2_PLACEMENT_3D('',#7945,#6418,#6419);
#5756=AXIS2_PLACEMENT_3D('',#7946,#6420,#6421);
#5757=AXIS2_PLACEMENT_3D('',#7949,#6424,#6425);
#5758=AXIS2_PLACEMENT_3D('',#7950,#6426,#6427);
#5759=AXIS2_PLACEMENT_3D('',#7951,#6428,#6429);
#5760=AXIS2_PLACEMENT_3D('',#7960,#6434,#6435);
#5761=AXIS2_PLACEMENT_3D('',#7966,#6439,#6440);
#5762=AXIS2_PLACEMENT_3D('',#7972,#6444,#6445);
#5763=AXIS2_PLACEMENT_3D('',#7978,#6449,#6450);
#5764=AXIS2_PLACEMENT_3D('',#7984,#6454,#6455);
#5765=AXIS2_PLACEMENT_3D('',#7987,#6458,#6459);
#5766=AXIS2_PLACEMENT_3D('',#7988,#6460,#6461);
#5767=AXIS2_PLACEMENT_3D('',#7989,#6462,#6463);
#5768=AXIS2_PLACEMENT_3D('',#7998,#6468,#6469);
#5769=AXIS2_PLACEMENT_3D('',#8004,#6473,#6474);
#5770=AXIS2_PLACEMENT_3D('',#8010,#6478,#6479);
#5771=AXIS2_PLACEMENT_3D('',#8016,#6483,#6484);
#5772=AXIS2_PLACEMENT_3D('',#8022,#6488,#6489);
#5773=AXIS2_PLACEMENT_3D('',#8025,#6492,#6493);
#5774=AXIS2_PLACEMENT_3D('',#8026,#6494,#6495);
#5775=AXIS2_PLACEMENT_3D('',#8027,#6496,#6497);
#5776=AXIS2_PLACEMENT_3D('',#8036,#6502,#6503);
#5777=AXIS2_PLACEMENT_3D('',#8042,#6507,#6508);
#5778=AXIS2_PLACEMENT_3D('',#8048,#6512,#6513);
#5779=AXIS2_PLACEMENT_3D('',#8054,#6517,#6518);
#5780=AXIS2_PLACEMENT_3D('',#8060,#6522,#6523);
#5781=AXIS2_PLACEMENT_3D('',#8063,#6526,#6527);
#5782=AXIS2_PLACEMENT_3D('',#8064,#6528,#6529);
#6224=DIRECTION('axis',(0.,0.,1.));
#6225=DIRECTION('refdir',(1.,0.,0.));
#6226=DIRECTION('center_axis',(0.,-1.,0.));
#6227=DIRECTION('ref_axis',(0.,0.,-1.));
#6228=DIRECTION('center_axis',(0.,1.,0.));
#6229=DIRECTION('ref_axis',(0.,0.,1.));
#6230=DIRECTION('',(0.,-1.,0.));
#6231=DIRECTION('center_axis',(-1.30104260698261E-16,1.,0.));
#6232=DIRECTION('ref_axis',(-1.,-1.30104260698261E-16,0.));
#6233=DIRECTION('center_axis',(0.,-1.,0.));
#6234=DIRECTION('ref_axis',(0.,0.,-1.));
#6235=DIRECTION('center_axis',(0.,1.,0.));
#6236=DIRECTION('ref_axis',(0.,0.,1.));
#6237=DIRECTION('',(0.,-1.,0.));
#6238=DIRECTION('center_axis',(-1.30104260698261E-16,1.,0.));
#6239=DIRECTION('ref_axis',(-1.,-1.30104260698261E-16,0.));
#6240=DIRECTION('center_axis',(0.,-1.,0.));
#6241=DIRECTION('ref_axis',(0.,0.,-1.));
#6242=DIRECTION('center_axis',(0.,1.,0.));
#6243=DIRECTION('ref_axis',(0.,0.,1.));
#6244=DIRECTION('',(0.,-1.,0.));
#6245=DIRECTION('center_axis',(-1.30104260698261E-16,1.,0.));
#6246=DIRECTION('ref_axis',(-1.,-1.30104260698261E-16,0.));
#6247=DIRECTION('center_axis',(0.,-1.,0.));
#6248=DIRECTION('ref_axis',(0.,0.,-1.));
#6249=DIRECTION('center_axis',(0.,1.,0.));
#6250=DIRECTION('ref_axis',(0.,0.,1.));
#6251=DIRECTION('',(0.,-1.,0.));
#6252=DIRECTION('center_axis',(-1.30104260698261E-16,1.,0.));
#6253=DIRECTION('ref_axis',(-1.,-1.30104260698261E-16,0.));
#6254=DIRECTION('center_axis',(0.,-1.,0.));
#6255=DIRECTION('ref_axis',(0.,0.,-1.));
#6256=DIRECTION('center_axis',(0.,1.,0.));
#6257=DIRECTION('ref_axis',(0.,0.,1.));
#6258=DIRECTION('',(0.,-1.,0.));
#6259=DIRECTION('center_axis',(-1.30104260698261E-16,1.,0.));
#6260=DIRECTION('ref_axis',(-1.,-1.30104260698261E-16,0.));
#6261=DIRECTION('center_axis',(0.,-1.,0.));
#6262=DIRECTION('ref_axis',(0.,0.,-1.));
#6263=DIRECTION('center_axis',(0.,1.,0.));
#6264=DIRECTION('ref_axis',(0.,0.,1.));
#6265=DIRECTION('',(0.,-1.,0.));
#6266=DIRECTION('center_axis',(-1.30104260698261E-16,1.,0.));
#6267=DIRECTION('ref_axis',(-1.,-1.30104260698261E-16,0.));
#6268=DIRECTION('center_axis',(0.,-1.,0.));
#6269=DIRECTION('ref_axis',(0.,0.,-1.));
#6270=DIRECTION('center_axis',(0.,1.,0.));
#6271=DIRECTION('ref_axis',(0.,0.,1.));
#6272=DIRECTION('',(0.,-1.,0.));
#6273=DIRECTION('center_axis',(-1.30104260698261E-16,1.,0.));
#6274=DIRECTION('ref_axis',(-1.,-1.30104260698261E-16,0.));
#6275=DIRECTION('center_axis',(0.,-1.,0.));
#6276=DIRECTION('ref_axis',(0.,0.,-1.));
#6277=DIRECTION('center_axis',(0.,1.,0.));
#6278=DIRECTION('ref_axis',(0.,0.,1.));
#6279=DIRECTION('',(0.,-1.,0.));
#6280=DIRECTION('center_axis',(-1.30104260698261E-16,1.,0.));
#6281=DIRECTION('ref_axis',(-1.,-1.30104260698261E-16,0.));
#6282=DIRECTION('',(0.,-1.,0.));
#6283=DIRECTION('center_axis',(0.258819045102518,0.,0.965925826289069));
#6284=DIRECTION('ref_axis',(0.965925826289069,0.,-0.258819045102518));
#6285=DIRECTION('',(-0.965925826289069,-1.25671065518696E-16,0.258819045102518));
#6286=DIRECTION('',(0.,-1.,0.));
#6287=DIRECTION('',(-0.965925826289069,0.,0.258819045102518));
#6288=DIRECTION('center_axis',(0.,-1.,0.));
#6289=DIRECTION('ref_axis',(0.,0.,-1.));
#6290=DIRECTION('center_axis',(-1.30104260698261E-16,1.,0.));
#6291=DIRECTION('ref_axis',(-1.,-1.30104260698261E-16,0.));
#6292=DIRECTION('',(0.,-1.,0.));
#6293=DIRECTION('center_axis',(0.,1.,0.));
#6294=DIRECTION('ref_axis',(0.,0.,-1.));
#6295=DIRECTION('center_axis',(1.,0.,0.));
#6296=DIRECTION('ref_axis',(0.,0.,-1.));
#6297=DIRECTION('',(0.,0.,1.));
#6298=DIRECTION('',(0.,-1.,0.));
#6299=DIRECTION('',(0.,0.,1.));
#6300=DIRECTION('center_axis',(0.,-1.,0.));
#6301=DIRECTION('ref_axis',(0.,0.,-1.));
#6302=DIRECTION('center_axis',(-1.30104260698261E-16,1.,0.));
#6303=DIRECTION('ref_axis',(-1.,-1.30104260698261E-16,0.));
#6304=DIRECTION('',(0.,-1.,0.));
#6305=DIRECTION('center_axis',(0.,1.,0.));
#6306=DIRECTION('ref_axis',(0.,0.,1.));
#6307=DIRECTION('center_axis',(0.258819045102518,0.,-0.965925826289069));
#6308=DIRECTION('ref_axis',(-0.965925826289069,0.,-0.258819045102518));
#6309=DIRECTION('',(0.965925826289069,1.25671065518696E-16,0.258819045102518));
#6310=DIRECTION('',(0.,-1.,0.));
#6311=DIRECTION('',(0.965925826289069,0.,0.258819045102518));
#6312=DIRECTION('center_axis',(0.,-1.,0.));
#6313=DIRECTION('ref_axis',(0.608761429008724,0.,0.793353340291233));
#6314=DIRECTION('center_axis',(-1.30104260698261E-16,1.,0.));
#6315=DIRECTION('ref_axis',(-1.,-1.30104260698261E-16,0.));
#6316=DIRECTION('',(0.,-1.,0.));
#6317=DIRECTION('center_axis',(0.,1.,0.));
#6318=DIRECTION('ref_axis',(0.,0.,1.));
#6319=DIRECTION('center_axis',(-1.,0.,0.));
#6320=DIRECTION('ref_axis',(0.,0.,1.));
#6321=DIRECTION('',(0.,0.,1.));
#6322=DIRECTION('',(0.,0.,-1.));
#6323=DIRECTION('center_axis',(0.,1.,0.));
#6324=DIRECTION('ref_axis',(0.,0.,1.));
#6325=DIRECTION('center_axis',(-1.30104260698261E-16,1.,0.));
#6326=DIRECTION('ref_axis',(-1.,-1.30104260698261E-16,0.));
#6327=DIRECTION('center_axis',(0.,-1.,0.));
#6328=DIRECTION('ref_axis',(0.,0.,-1.));
#6329=DIRECTION('center_axis',(0.,-1.,0.));
#6330=DIRECTION('ref_axis',(0.,0.,-1.));
#6331=DIRECTION('',(0.,-1.,0.));
#6332=DIRECTION('center_axis',(0.,1.,0.));
#6333=DIRECTION('ref_axis',(0.,0.,1.));
#6334=DIRECTION('center_axis',(0.,-1.,0.));
#6335=DIRECTION('ref_axis',(0.,0.,-1.));
#6336=DIRECTION('center_axis',(0.,-1.,0.));
#6337=DIRECTION('ref_axis',(0.,0.,-1.));
#6338=DIRECTION('',(0.,-1.,0.));
#6339=DIRECTION('center_axis',(0.,1.,0.));
#6340=DIRECTION('ref_axis',(0.,0.,1.));
#6341=DIRECTION('center_axis',(0.,-1.,0.));
#6342=DIRECTION('ref_axis',(0.,0.,-1.));
#6343=DIRECTION('center_axis',(0.,-1.,0.));
#6344=DIRECTION('ref_axis',(0.,0.,-1.));
#6345=DIRECTION('',(0.,-1.,0.));
#6346=DIRECTION('center_axis',(0.,1.,0.));
#6347=DIRECTION('ref_axis',(0.,0.,1.));
#6348=DIRECTION('center_axis',(0.,-1.,0.));
#6349=DIRECTION('ref_axis',(0.,0.,-1.));
#6350=DIRECTION('center_axis',(0.,-1.,0.));
#6351=DIRECTION('ref_axis',(0.,0.,-1.));
#6352=DIRECTION('',(0.,-1.,0.));
#6353=DIRECTION('center_axis',(0.,1.,0.));
#6354=DIRECTION('ref_axis',(0.,0.,1.));
#6355=DIRECTION('center_axis',(0.,-1.,0.));
#6356=DIRECTION('ref_axis',(0.,0.,-1.));
#6357=DIRECTION('center_axis',(0.,-1.,0.));
#6358=DIRECTION('ref_axis',(0.,0.,-1.));
#6359=DIRECTION('',(0.,-1.,0.));
#6360=DIRECTION('center_axis',(0.,1.,0.));
#6361=DIRECTION('ref_axis',(0.,0.,1.));
#6362=DIRECTION('',(0.,-1.,0.));
#6363=DIRECTION('center_axis',(0.,-1.,0.));
#6364=DIRECTION('ref_axis',(0.,0.,-1.));
#6365=DIRECTION('center_axis',(0.,-1.,0.));
#6366=DIRECTION('ref_axis',(0.,0.,-1.));
#6367=DIRECTION('',(0.,-1.,0.));
#6368=DIRECTION('center_axis',(0.,1.,0.));
#6369=DIRECTION('ref_axis',(0.,0.,1.));
#6370=DIRECTION('center_axis',(0.,-1.,0.));
#6371=DIRECTION('ref_axis',(0.,0.,-1.));
#6372=DIRECTION('center_axis',(0.,-1.,0.));
#6373=DIRECTION('ref_axis',(0.,0.,-1.));
#6374=DIRECTION('',(0.,-1.,0.));
#6375=DIRECTION('center_axis',(0.,1.,0.));
#6376=DIRECTION('ref_axis',(0.,0.,1.));
#6377=DIRECTION('center_axis',(0.,-1.,0.));
#6378=DIRECTION('ref_axis',(0.,0.,-1.));
#6379=DIRECTION('center_axis',(0.,-1.,0.));
#6380=DIRECTION('ref_axis',(0.,0.,-1.));
#6381=DIRECTION('',(0.,-1.,0.));
#6382=DIRECTION('center_axis',(0.,1.,0.));
#6383=DIRECTION('ref_axis',(0.,0.,1.));
#6384=DIRECTION('center_axis',(-1.,0.,0.));
#6385=DIRECTION('ref_axis',(0.,0.,1.));
#6386=DIRECTION('',(0.,0.,1.));
#6387=DIRECTION('',(0.,-1.,0.));
#6388=DIRECTION('',(0.,0.,-1.));
#6389=DIRECTION('center_axis',(0.,-1.,0.));
#6390=DIRECTION('ref_axis',(0.608761429008723,0.,0.793353340291234));
#6391=DIRECTION('center_axis',(0.,-1.,0.));
#6392=DIRECTION('ref_axis',(0.,0.,-1.));
#6393=DIRECTION('',(0.,-1.,0.));
#6394=DIRECTION('center_axis',(0.,1.,0.));
#6395=DIRECTION('ref_axis',(0.,0.,1.));
#6396=DIRECTION('center_axis',(0.258819045102518,0.,-0.965925826289069));
#6397=DIRECTION('ref_axis',(-0.965925826289069,0.,-0.258819045102518));
#6398=DIRECTION('',(-0.965925826289069,0.,-0.258819045102518));
#6399=DIRECTION('',(0.,-1.,0.));
#6400=DIRECTION('',(0.965925826289069,0.,0.258819045102518));
#6401=DIRECTION('center_axis',(0.,-1.,0.));
#6402=DIRECTION('ref_axis',(0.,0.,-1.));
#6403=DIRECTION('center_axis',(0.,-1.,0.));
#6404=DIRECTION('ref_axis',(0.,0.,-1.));
#6405=DIRECTION('',(0.,-1.,0.));
#6406=DIRECTION('center_axis',(0.,1.,0.));
#6407=DIRECTION('ref_axis',(0.,0.,1.));
#6408=DIRECTION('center_axis',(1.,0.,0.));
#6409=DIRECTION('ref_axis',(0.,0.,-1.));
#6410=DIRECTION('',(0.,0.,1.));
#6411=DIRECTION('',(0.,-1.,0.));
#6412=DIRECTION('',(0.,0.,1.));
#6413=DIRECTION('center_axis',(0.,-1.,0.));
#6414=DIRECTION('ref_axis',(0.,0.,-1.));
#6415=DIRECTION('center_axis',(0.,-1.,0.));
#6416=DIRECTION('ref_axis',(0.,0.,-1.));
#6417=DIRECTION('',(0.,-1.,0.));
#6418=DIRECTION('center_axis',(0.,1.,0.));
#6419=DIRECTION('ref_axis',(0.,0.,-1.));
#6420=DIRECTION('center_axis',(0.258819045102518,0.,0.965925826289069));
#6421=DIRECTION('ref_axis',(0.965925826289069,0.,-0.258819045102518));
#6422=DIRECTION('',(0.965925826289069,0.,-0.258819045102518));
#6423=DIRECTION('',(-0.965925826289069,0.,0.258819045102518));
#6424=DIRECTION('center_axis',(0.,1.,0.));
#6425=DIRECTION('ref_axis',(0.,0.,1.));
#6426=DIRECTION('center_axis',(0.,-1.,0.));
#6427=DIRECTION('ref_axis',(0.,0.,-1.));
#6428=DIRECTION('center_axis',(0.499999999999999,0.,-0.866025403784439));
#6429=DIRECTION('ref_axis',(-0.866025403784439,0.,-0.499999999999999));
#6430=DIRECTION('',(0.866025403784439,0.,0.499999999999999));
#6431=DIRECTION('',(0.,-1.,0.));
#6432=DIRECTION('',(0.866025403784439,0.,0.499999999999999));
#6433=DIRECTION('',(0.,-1.,0.));
#6434=DIRECTION('center_axis',(-0.5,0.,-0.866025403784438));
#6435=DIRECTION('ref_axis',(-0.866025403784438,0.,0.5));
#6436=DIRECTION('',(0.866025403784438,0.,-0.5));
#6437=DIRECTION('',(0.,-1.,0.));
#6438=DIRECTION('',(0.866025403784438,0.,-0.5));
#6439=DIRECTION('center_axis',(-1.,0.,0.));
#6440=DIRECTION('ref_axis',(0.,0.,1.));
#6441=DIRECTION('',(0.,0.,-1.));
#6442=DIRECTION('',(0.,-1.,0.));
#6443=DIRECTION('',(0.,0.,-1.));
#6444=DIRECTION('center_axis',(-0.5,0.,0.866025403784439));
#6445=DIRECTION('ref_axis',(0.866025403784439,0.,0.5));
#6446=DIRECTION('',(-0.866025403784439,0.,-0.5));
#6447=DIRECTION('',(0.,-1.,0.));
#6448=DIRECTION('',(-0.866025403784439,0.,-0.5));
#6449=DIRECTION('center_axis',(0.5,0.,0.866025403784438));
#6450=DIRECTION('ref_axis',(0.866025403784438,0.,-0.5));
#6451=DIRECTION('',(-0.866025403784438,0.,0.5));
#6452=DIRECTION('',(0.,-1.,0.));
#6453=DIRECTION('',(-0.866025403784438,0.,0.5));
#6454=DIRECTION('center_axis',(1.,0.,0.));
#6455=DIRECTION('ref_axis',(0.,0.,-1.));
#6456=DIRECTION('',(0.,0.,1.));
#6457=DIRECTION('',(0.,0.,1.));
#6458=DIRECTION('center_axis',(0.,1.,0.));
#6459=DIRECTION('ref_axis',(0.,0.,1.));
#6460=DIRECTION('center_axis',(0.,1.,0.));
#6461=DIRECTION('ref_axis',(0.,0.,1.));
#6462=DIRECTION('center_axis',(0.866025403784438,0.,-0.500000000000002));
#6463=DIRECTION('ref_axis',(-0.500000000000002,0.,-0.866025403784437));
#6464=DIRECTION('',(0.500000000000002,0.,0.866025403784437));
#6465=DIRECTION('',(0.,-1.,0.));
#6466=DIRECTION('',(0.500000000000002,0.,0.866025403784437));
#6467=DIRECTION('',(0.,-1.,0.));
#6468=DIRECTION('center_axis',(0.,0.,-1.));
#6469=DIRECTION('ref_axis',(-1.,0.,0.));
#6470=DIRECTION('',(1.,0.,0.));
#6471=DIRECTION('',(0.,-1.,0.));
#6472=DIRECTION('',(1.,0.,0.));
#6473=DIRECTION('center_axis',(-0.866025403784436,0.,-0.500000000000005));
#6474=DIRECTION('ref_axis',(-0.500000000000005,0.,0.866025403784436));
#6475=DIRECTION('',(0.500000000000004,0.,-0.866025403784436));
#6476=DIRECTION('',(0.,-1.,0.));
#6477=DIRECTION('',(0.500000000000004,0.,-0.866025403784436));
#6478=DIRECTION('center_axis',(-0.866025403784438,0.,0.500000000000002));
#6479=DIRECTION('ref_axis',(0.500000000000002,0.,0.866025403784437));
#6480=DIRECTION('',(-0.500000000000002,0.,-0.866025403784438));
#6481=DIRECTION('',(0.,-1.,0.));
#6482=DIRECTION('',(-0.500000000000002,0.,-0.866025403784438));
#6483=DIRECTION('center_axis',(0.,0.,1.));
#6484=DIRECTION('ref_axis',(1.,0.,0.));
#6485=DIRECTION('',(-1.,0.,0.));
#6486=DIRECTION('',(0.,-1.,0.));
#6487=DIRECTION('',(-1.,0.,0.));
#6488=DIRECTION('center_axis',(0.866025403784439,0.,0.5));
#6489=DIRECTION('ref_axis',(0.5,0.,-0.866025403784439));
#6490=DIRECTION('',(-0.5,0.,0.866025403784439));
#6491=DIRECTION('',(-0.5,0.,0.866025403784439));
#6492=DIRECTION('center_axis',(0.,1.,0.));
#6493=DIRECTION('ref_axis',(0.,0.,1.));
#6494=DIRECTION('center_axis',(0.,1.,0.));
#6495=DIRECTION('ref_axis',(0.,0.,1.));
#6496=DIRECTION('center_axis',(-0.5,0.,-0.866025403784439));
#6497=DIRECTION('ref_axis',(-0.866025403784439,0.,0.5));
#6498=DIRECTION('',(0.866025403784439,0.,-0.5));
#6499=DIRECTION('',(0.,-1.,0.));
#6500=DIRECTION('',(0.866025403784439,0.,-0.5));
#6501=DIRECTION('',(0.,-1.,0.));
#6502=DIRECTION('center_axis',(-1.,0.,0.));
#6503=DIRECTION('ref_axis',(0.,0.,1.));
#6504=DIRECTION('',(0.,0.,-1.));
#6505=DIRECTION('',(0.,-1.,0.));
#6506=DIRECTION('',(0.,0.,-1.));
#6507=DIRECTION('center_axis',(-0.5,0.,0.866025403784439));
#6508=DIRECTION('ref_axis',(0.866025403784439,0.,0.5));
#6509=DIRECTION('',(-0.866025403784439,0.,-0.5));
#6510=DIRECTION('',(0.,-1.,0.));
#6511=DIRECTION('',(-0.866025403784439,0.,-0.5));
#6512=DIRECTION('center_axis',(0.499999999999999,0.,0.866025403784439));
#6513=DIRECTION('ref_axis',(0.866025403784439,0.,-0.499999999999999));
#6514=DIRECTION('',(-0.866025403784439,0.,0.499999999999999));
#6515=DIRECTION('',(0.,-1.,0.));
#6516=DIRECTION('',(-0.866025403784439,0.,0.499999999999999));
#6517=DIRECTION('center_axis',(1.,0.,0.));
#6518=DIRECTION('ref_axis',(0.,0.,-1.));
#6519=DIRECTION('',(0.,0.,1.));
#6520=DIRECTION('',(0.,-1.,0.));
#6521=DIRECTION('',(0.,0.,1.));
#6522=DIRECTION('center_axis',(0.499999999999998,0.,-0.86602540378444));
#6523=DIRECTION('ref_axis',(-0.86602540378444,0.,-0.499999999999998));
#6524=DIRECTION('',(0.86602540378444,0.,0.499999999999998));
#6525=DIRECTION('',(0.86602540378444,0.,0.499999999999998));
#6526=DIRECTION('center_axis',(0.,1.,0.));
#6527=DIRECTION('ref_axis',(0.,0.,1.));
#6528=DIRECTION('center_axis',(0.,1.,0.));
#6529=DIRECTION('ref_axis',(0.,0.,1.));
#7766=CARTESIAN_POINT('',(0.,0.,0.));
#7767=CARTESIAN_POINT('Origin',(72.,22.,-30.));
#7768=CARTESIAN_POINT('',(72.,22.,-28.));
#7769=CARTESIAN_POINT('Origin',(72.,22.,-30.));
#7770=CARTESIAN_POINT('',(72.,19.,-28.));
#7771=CARTESIAN_POINT('',(72.,22.,-28.));
#7772=CARTESIAN_POINT('Origin',(72.,19.,-30.));
#7773=CARTESIAN_POINT('Origin',(72.,22.,30.));
#7774=CARTESIAN_POINT('',(72.,22.,32.));
#7775=CARTESIAN_POINT('Origin',(72.,22.,30.));
#7776=CARTESIAN_POINT('',(72.,19.,32.));
#7777=CARTESIAN_POINT('',(72.,22.,32.));
#7778=CARTESIAN_POINT('Origin',(72.,19.,30.));
#7779=CARTESIAN_POINT('Origin',(7.,22.,0.));
#7780=CARTESIAN_POINT('',(7.,22.,2.));
#7781=CARTESIAN_POINT('Origin',(7.,22.,0.));
#7782=CARTESIAN_POINT('',(7.,19.,2.));
#7783=CARTESIAN_POINT('',(7.,22.,2.));
#7784=CARTESIAN_POINT('Origin',(7.,19.,0.));
#7785=CARTESIAN_POINT('Origin',(42.,22.,18.));
#7786=CARTESIAN_POINT('',(42.,22.,20.5));
#7787=CARTESIAN_POINT('Origin',(42.,22.,18.));
#7788=CARTESIAN_POINT('',(42.,19.,20.5));
#7789=CARTESIAN_POINT('',(42.,22.,20.5));
#7790=CARTESIAN_POINT('Origin',(42.,19.,18.));
#7791=CARTESIAN_POINT('Origin',(42.,22.,-18.));
#7792=CARTESIAN_POINT('',(42.,22.,-15.5));
#7793=CARTESIAN_POINT('Origin',(42.,22.,-18.));
#7794=CARTESIAN_POINT('',(42.,19.,-15.5));
#7795=CARTESIAN_POINT('',(42.,22.,-15.5));
#7796=CARTESIAN_POINT('Origin',(42.,19.,-18.));
#7797=CARTESIAN_POINT('Origin',(12.,22.,12.5));
#7798=CARTESIAN_POINT('',(12.,22.,15.));
#7799=CARTESIAN_POINT('Origin',(12.,22.,12.5));
#7800=CARTESIAN_POINT('',(12.,19.,15.));
#7801=CARTESIAN_POINT('',(12.,22.,15.));
#7802=CARTESIAN_POINT('Origin',(12.,19.,12.5));
#7803=CARTESIAN_POINT('Origin',(12.,22.,-12.5));
#7804=CARTESIAN_POINT('',(12.,22.,-10.));
#7805=CARTESIAN_POINT('Origin',(12.,22.,-12.5));
#7806=CARTESIAN_POINT('',(12.,19.,-10.));
#7807=CARTESIAN_POINT('',(12.,22.,-10.));
#7808=CARTESIAN_POINT('Origin',(12.,19.,-12.5));
#7809=CARTESIAN_POINT('Origin',(72.,22.,-33.51013241176));
#7810=CARTESIAN_POINT('',(80.,22.,-33.51013241176));
#7811=CARTESIAN_POINT('',(69.9294476391799,22.,-41.2375390220725));
#7812=CARTESIAN_POINT('Origin',(72.,22.,-33.51013241176));
#7813=CARTESIAN_POINT('',(80.,19.,-33.51013241176));
#7814=CARTESIAN_POINT('',(80.,22.,-33.51013241176));
#7815=CARTESIAN_POINT('',(69.9294476391799,19.,-41.2375390220725));
#7816=CARTESIAN_POINT('Origin',(72.,19.,-33.51013241176));
#7817=CARTESIAN_POINT('',(69.9294476391799,22.,-41.2375390220725));
#7818=CARTESIAN_POINT('Origin',(69.9294476391799,22.,-41.2375390220725));
#7819=CARTESIAN_POINT('',(5.92944763917986,19.,-24.0887907064809));
#7820=CARTESIAN_POINT('',(69.9294476391799,19.,-41.2375390220725));
#7821=CARTESIAN_POINT('',(5.92944763917986,22.,-24.0887907064809));
#7822=CARTESIAN_POINT('',(5.92944763917986,22.,-24.0887907064809));
#7823=CARTESIAN_POINT('',(69.9294476391799,22.,-41.2375390220725));
#7824=CARTESIAN_POINT('Origin',(8.,22.,-16.3613840961683));
#7825=CARTESIAN_POINT('',(8.57252759403147E-16,19.,-16.3613840961683));
#7826=CARTESIAN_POINT('Origin',(8.,19.,-16.3613840961683));
#7827=CARTESIAN_POINT('',(3.46944695195361E-15,22.,-16.3613840961683));
#7828=CARTESIAN_POINT('',(3.46944695195361E-15,22.,-16.3613840961683));
#7829=CARTESIAN_POINT('Origin',(8.,22.,-16.3613840961683));
#7830=CARTESIAN_POINT('Origin',(3.46944695195361E-15,22.,-16.3613840961683));
#7831=CARTESIAN_POINT('',(3.46944695195361E-15,19.,16.3613840961683));
#7832=CARTESIAN_POINT('',(8.57252759403147E-16,19.,-50.));
#7833=CARTESIAN_POINT('',(3.46944695195361E-15,22.,16.3613840961683));
#7834=CARTESIAN_POINT('',(3.46944695195361E-15,22.,16.3613840961683));
#7835=CARTESIAN_POINT('',(3.46944695195361E-15,22.,-16.3613840961683));
#7836=CARTESIAN_POINT('Origin',(8.,22.,16.3613840961683));
#7837=CARTESIAN_POINT('',(5.92944763917986,19.,24.0887907064809));
#7838=CARTESIAN_POINT('Origin',(8.,19.,16.3613840961683));
#7839=CARTESIAN_POINT('',(5.92944763917986,22.,24.0887907064809));
#7840=CARTESIAN_POINT('',(5.92944763917986,22.,24.0887907064809));
#7841=CARTESIAN_POINT('Origin',(8.,22.,16.3613840961683));
#7842=CARTESIAN_POINT('Origin',(5.92944763917986,22.,24.0887907064809));
#7843=CARTESIAN_POINT('',(69.9294476391799,19.,41.2375390220725));
#7844=CARTESIAN_POINT('',(5.92944763917986,19.,24.0887907064809));
#7845=CARTESIAN_POINT('',(69.9294476391799,22.,41.2375390220725));
#7846=CARTESIAN_POINT('',(69.9294476391799,22.,41.2375390220725));
#7847=CARTESIAN_POINT('',(5.92944763917986,22.,24.0887907064809));
#7848=CARTESIAN_POINT('Origin',(72.,22.,33.51013241176));
#7849=CARTESIAN_POINT('',(80.,19.,33.5101324117599));
#7850=CARTESIAN_POINT('Origin',(72.,19.,33.51013241176));
#7851=CARTESIAN_POINT('',(80.,22.,33.51013241176));
#7852=CARTESIAN_POINT('',(80.,22.,33.51013241176));
#7853=CARTESIAN_POINT('Origin',(72.,22.,33.51013241176));
#7854=CARTESIAN_POINT('Origin',(80.,22.,33.51013241176));
#7855=CARTESIAN_POINT('',(80.,19.,-50.));
#7856=CARTESIAN_POINT('',(80.,22.,33.51013241176));
#7857=CARTESIAN_POINT('Origin',(72.,22.,-33.51013241176));
#7858=CARTESIAN_POINT('Origin',(8.57252759403147E-16,19.,-50.));
#7859=CARTESIAN_POINT('Origin',(72.,22.,-30.));
#7860=CARTESIAN_POINT('',(72.,3.,-28.));
#7861=CARTESIAN_POINT('Origin',(72.,3.,-30.));
#7862=CARTESIAN_POINT('',(72.,0.,-28.));
#7863=CARTESIAN_POINT('',(72.,22.,-28.));
#7864=CARTESIAN_POINT('Origin',(72.,0.,-30.));
#7865=CARTESIAN_POINT('Origin',(72.,22.,30.));
#7866=CARTESIAN_POINT('',(72.,3.,32.));
#7867=CARTESIAN_POINT('Origin',(72.,3.,30.));
#7868=CARTESIAN_POINT('',(72.,0.,32.));
#7869=CARTESIAN_POINT('',(72.,22.,32.));
#7870=CARTESIAN_POINT('Origin',(72.,0.,30.));
#7871=CARTESIAN_POINT('Origin',(42.,22.,18.));
#7872=CARTESIAN_POINT('',(42.,3.,20.5));
#7873=CARTESIAN_POINT('Origin',(42.,3.,18.));
#7874=CARTESIAN_POINT('',(42.,0.,20.5));
#7875=CARTESIAN_POINT('',(42.,22.,20.5));
#7876=CARTESIAN_POINT('Origin',(42.,0.,18.));
#7877=CARTESIAN_POINT('Origin',(12.,22.,12.5));
#7878=CARTESIAN_POINT('',(12.,3.,15.));
#7879=CARTESIAN_POINT('Origin',(12.,3.,12.5));
#7880=CARTESIAN_POINT('',(12.,0.,15.));
#7881=CARTESIAN_POINT('',(12.,22.,15.));
#7882=CARTESIAN_POINT('Origin',(12.,0.,12.5));
#7883=CARTESIAN_POINT('Origin',(72.,22.,-33.51013241176));
#7884=CARTESIAN_POINT('',(69.9294476391799,3.,-41.2375390220725));
#7885=CARTESIAN_POINT('',(80.,3.,-33.51013241176));
#7886=CARTESIAN_POINT('Origin',(72.,3.,-33.51013241176));
#7887=CARTESIAN_POINT('',(80.,0.,-33.51013241176));
#7888=CARTESIAN_POINT('',(80.,22.,-33.51013241176));
#7889=CARTESIAN_POINT('',(69.9294476391799,0.,-41.2375390220725));
#7890=CARTESIAN_POINT('Origin',(72.,0.,-33.51013241176));
#7891=CARTESIAN_POINT('',(69.9294476391799,22.,-41.2375390220725));
#7892=CARTESIAN_POINT('Origin',(12.,22.,-12.5));
#7893=CARTESIAN_POINT('',(12.,3.,-10.));
#7894=CARTESIAN_POINT('Origin',(12.,3.,-12.5));
#7895=CARTESIAN_POINT('',(12.,0.,-10.));
#7896=CARTESIAN_POINT('',(12.,22.,-10.));
#7897=CARTESIAN_POINT('Origin',(12.,0.,-12.5));
#7898=CARTESIAN_POINT('Origin',(42.,22.,-18.));
#7899=CARTESIAN_POINT('',(42.,3.,-15.5));
#7900=CARTESIAN_POINT('Origin',(42.,3.,-18.));
#7901=CARTESIAN_POINT('',(42.,0.,-15.5));
#7902=CARTESIAN_POINT('',(42.,22.,-15.5));
#7903=CARTESIAN_POINT('Origin',(42.,0.,-18.));
#7904=CARTESIAN_POINT('Origin',(7.,22.,0.));
#7905=CARTESIAN_POINT('',(7.,3.,2.));
#7906=CARTESIAN_POINT('Origin',(7.,3.,0.));
#7907=CARTESIAN_POINT('',(7.,0.,2.));
#7908=CARTESIAN_POINT('',(7.,22.,2.));
#7909=CARTESIAN_POINT('Origin',(7.,0.,0.));
#7910=CARTESIAN_POINT('Origin',(80.,22.,33.51013241176));
#7911=CARTESIAN_POINT('',(80.,3.,33.51013241176));
#7912=CARTESIAN_POINT('',(80.,3.,-50.));
#7913=CARTESIAN_POINT('',(80.,0.,33.51013241176));
#7914=CARTESIAN_POINT('',(80.,22.,33.51013241176));
#7915=CARTESIAN_POINT('',(80.,0.,33.51013241176));
#7916=CARTESIAN_POINT('Origin',(72.,22.,33.51013241176));
#7917=CARTESIAN_POINT('',(69.9294476391799,3.,41.2375390220725));
#7918=CARTESIAN_POINT('Origin',(72.,3.,33.51013241176));
#7919=CARTESIAN_POINT('',(69.9294476391799,0.,41.2375390220725));
#7920=CARTESIAN_POINT('',(69.9294476391799,22.,41.2375390220725));
#7921=CARTESIAN_POINT('Origin',(72.,0.,33.51013241176));
#7922=CARTESIAN_POINT('Origin',(5.92944763917986,22.,24.0887907064809));
#7923=CARTESIAN_POINT('',(5.92944763917986,3.,24.0887907064809));
#7924=CARTESIAN_POINT('',(5.92944763917986,3.,24.0887907064809));
#7925=CARTESIAN_POINT('',(5.92944763917986,0.,24.0887907064809));
#7926=CARTESIAN_POINT('',(5.92944763917986,22.,24.0887907064809));
#7927=CARTESIAN_POINT('',(5.92944763917986,0.,24.0887907064809));
#7928=CARTESIAN_POINT('Origin',(8.,22.,16.3613840961683));
#7929=CARTESIAN_POINT('',(5.20417042793042E-15,3.,16.3613840961683));
#7930=CARTESIAN_POINT('Origin',(8.,3.,16.3613840961683));
#7931=CARTESIAN_POINT('',(3.46944695195361E-15,0.,16.3613840961683));
#7932=CARTESIAN_POINT('',(3.46944695195361E-15,22.,16.3613840961683));
#7933=CARTESIAN_POINT('Origin',(8.,0.,16.3613840961683));
#7934=CARTESIAN_POINT('Origin',(3.46944695195361E-15,22.,-16.3613840961683));
#7935=CARTESIAN_POINT('',(1.83697019872103E-15,3.,-16.3613840961683));
#7936=CARTESIAN_POINT('',(1.83697019872103E-15,3.,-50.));
#7937=CARTESIAN_POINT('',(3.46944695195361E-15,0.,-16.3613840961683));
#7938=CARTESIAN_POINT('',(3.46944695195361E-15,22.,-16.3613840961683));
#7939=CARTESIAN_POINT('',(3.46944695195361E-15,0.,-16.3613840961683));
#7940=CARTESIAN_POINT('Origin',(8.,22.,-16.3613840961683));
#7941=CARTESIAN_POINT('',(5.92944763917986,3.,-24.0887907064809));
#7942=CARTESIAN_POINT('Origin',(8.,3.,-16.3613840961683));
#7943=CARTESIAN_POINT('',(5.92944763917986,0.,-24.0887907064809));
#7944=CARTESIAN_POINT('',(5.92944763917986,22.,-24.0887907064809));
#7945=CARTESIAN_POINT('Origin',(8.,0.,-16.3613840961683));
#7946=CARTESIAN_POINT('Origin',(69.9294476391799,22.,-41.2375390220725));
#7947=CARTESIAN_POINT('',(69.9294476391799,3.,-41.2375390220725));
#7948=CARTESIAN_POINT('',(69.9294476391799,0.,-41.2375390220725));
#7949=CARTESIAN_POINT('Origin',(72.,0.,-33.51013241176));
#7950=CARTESIAN_POINT('Origin',(1.83697019872103E-15,3.,-50.));
#7951=CARTESIAN_POINT('Origin',(5.,19.,1.15470053837925));
#7952=CARTESIAN_POINT('',(5.,3.,1.15470053837925));
#7953=CARTESIAN_POINT('',(7.00000000000001,3.,2.3094010767585));
#7954=CARTESIAN_POINT('',(5.,3.,1.15470053837925));
#7955=CARTESIAN_POINT('',(7.00000000000001,19.,2.3094010767585));
#7956=CARTESIAN_POINT('',(7.00000000000001,19.,2.3094010767585));
#7957=CARTESIAN_POINT('',(5.,19.,1.15470053837925));
#7958=CARTESIAN_POINT('',(5.,19.,1.15470053837925));
#7959=CARTESIAN_POINT('',(5.,19.,1.15470053837925));
#7960=CARTESIAN_POINT('Origin',(7.00000000000001,19.,2.3094010767585));
#7961=CARTESIAN_POINT('',(9.00000000000001,3.,1.15470053837925));
#7962=CARTESIAN_POINT('',(7.00000000000001,3.,2.3094010767585));
#7963=CARTESIAN_POINT('',(9.00000000000001,19.,1.15470053837925));
#7964=CARTESIAN_POINT('',(9.00000000000001,19.,1.15470053837925));
#7965=CARTESIAN_POINT('',(7.00000000000001,19.,2.3094010767585));
#7966=CARTESIAN_POINT('Origin',(9.00000000000001,19.,1.15470053837925));
#7967=CARTESIAN_POINT('',(9.00000000000001,3.,-1.15470053837925));
#7968=CARTESIAN_POINT('',(9.00000000000001,3.,1.15470053837925));
#7969=CARTESIAN_POINT('',(9.00000000000001,19.,-1.15470053837925));
#7970=CARTESIAN_POINT('',(9.00000000000001,19.,-1.15470053837925));
#7971=CARTESIAN_POINT('',(9.00000000000001,19.,1.15470053837925));
#7972=CARTESIAN_POINT('Origin',(9.00000000000001,19.,-1.15470053837925));
#7973=CARTESIAN_POINT('',(7.,3.,-2.30940107675851));
#7974=CARTESIAN_POINT('',(9.00000000000001,3.,-1.15470053837925));
#7975=CARTESIAN_POINT('',(7.,19.,-2.30940107675851));
#7976=CARTESIAN_POINT('',(7.,19.,-2.30940107675851));
#7977=CARTESIAN_POINT('',(9.00000000000001,19.,-1.15470053837925));
#7978=CARTESIAN_POINT('Origin',(7.,19.,-2.30940107675851));
#7979=CARTESIAN_POINT('',(5.,3.,-1.15470053837925));
#7980=CARTESIAN_POINT('',(7.,3.,-2.30940107675851));
#7981=CARTESIAN_POINT('',(5.,19.,-1.15470053837925));
#7982=CARTESIAN_POINT('',(5.,19.,-1.15470053837925));
#7983=CARTESIAN_POINT('',(7.,19.,-2.30940107675851));
#7984=CARTESIAN_POINT('Origin',(5.,19.,-1.15470053837925));
#7985=CARTESIAN_POINT('',(5.,3.,-1.15470053837925));
#7986=CARTESIAN_POINT('',(5.,19.,-1.15470053837925));
#7987=CARTESIAN_POINT('Origin',(7.00000000000001,19.,2.3094010767585));
#7988=CARTESIAN_POINT('Origin',(7.00000000000001,3.,2.3094010767585));
#7989=CARTESIAN_POINT('Origin',(69.6905989232415,19.,30.));
#7990=CARTESIAN_POINT('',(69.6905989232415,3.,30.));
#7991=CARTESIAN_POINT('',(70.8452994616208,3.,32.));
#7992=CARTESIAN_POINT('',(69.6905989232415,3.,30.));
#7993=CARTESIAN_POINT('',(70.8452994616208,19.,32.));
#7994=CARTESIAN_POINT('',(70.8452994616208,19.,32.));
#7995=CARTESIAN_POINT('',(69.6905989232415,19.,30.));
#7996=CARTESIAN_POINT('',(69.6905989232415,19.,30.));
#7997=CARTESIAN_POINT('',(69.6905989232415,19.,30.));
#7998=CARTESIAN_POINT('Origin',(70.8452994616208,19.,32.));
#7999=CARTESIAN_POINT('',(73.1547005383792,3.,32.));
#8000=CARTESIAN_POINT('',(70.8452994616208,3.,32.));
#8001=CARTESIAN_POINT('',(73.1547005383792,19.,32.));
#8002=CARTESIAN_POINT('',(73.1547005383792,19.,32.));
#8003=CARTESIAN_POINT('',(70.8452994616208,19.,32.));
#8004=CARTESIAN_POINT('Origin',(73.1547005383792,19.,32.));
#8005=CARTESIAN_POINT('',(74.3094010767585,3.,30.));
#8006=CARTESIAN_POINT('',(73.1547005383792,3.,32.));
#8007=CARTESIAN_POINT('',(74.3094010767585,19.,30.));
#8008=CARTESIAN_POINT('',(74.3094010767585,19.,30.));
#8009=CARTESIAN_POINT('',(73.1547005383792,19.,32.));
#8010=CARTESIAN_POINT('Origin',(74.3094010767585,19.,30.));
#8011=CARTESIAN_POINT('',(73.1547005383792,3.,28.));
#8012=CARTESIAN_POINT('',(74.3094010767585,3.,30.));
#8013=CARTESIAN_POINT('',(73.1547005383792,19.,28.));
#8014=CARTESIAN_POINT('',(73.1547005383792,19.,28.));
#8015=CARTESIAN_POINT('',(74.3094010767585,19.,30.));
#8016=CARTESIAN_POINT('Origin',(73.1547005383792,19.,28.));
#8017=CARTESIAN_POINT('',(70.8452994616208,3.,28.));
#8018=CARTESIAN_POINT('',(73.1547005383792,3.,28.));
#8019=CARTESIAN_POINT('',(70.8452994616208,19.,28.));
#8020=CARTESIAN_POINT('',(70.8452994616208,19.,28.));
#8021=CARTESIAN_POINT('',(73.1547005383792,19.,28.));
#8022=CARTESIAN_POINT('Origin',(70.8452994616208,19.,28.));
#8023=CARTESIAN_POINT('',(70.8452994616208,3.,28.));
#8024=CARTESIAN_POINT('',(70.8452994616208,19.,28.));
#8025=CARTESIAN_POINT('Origin',(70.8452994616208,19.,32.));
#8026=CARTESIAN_POINT('Origin',(70.8452994616208,3.,32.));
#8027=CARTESIAN_POINT('Origin',(72.0000000000001,19.,-27.6905989232415));
#8028=CARTESIAN_POINT('',(72.0000000000001,3.,-27.6905989232415));
#8029=CARTESIAN_POINT('',(74.,3.,-28.8452994616208));
#8030=CARTESIAN_POINT('',(72.0000000000001,3.,-27.6905989232415));
#8031=CARTESIAN_POINT('',(74.,19.,-28.8452994616208));
#8032=CARTESIAN_POINT('',(74.,19.,-28.8452994616208));
#8033=CARTESIAN_POINT('',(72.0000000000001,19.,-27.6905989232415));
#8034=CARTESIAN_POINT('',(72.0000000000001,19.,-27.6905989232415));
#8035=CARTESIAN_POINT('',(72.0000000000001,19.,-27.6905989232415));
#8036=CARTESIAN_POINT('Origin',(74.,19.,-28.8452994616208));
#8037=CARTESIAN_POINT('',(74.,3.,-31.1547005383792));
#8038=CARTESIAN_POINT('',(74.,3.,-28.8452994616208));
#8039=CARTESIAN_POINT('',(74.,19.,-31.1547005383792));
#8040=CARTESIAN_POINT('',(74.,19.,-31.1547005383792));
#8041=CARTESIAN_POINT('',(74.,19.,-28.8452994616208));
#8042=CARTESIAN_POINT('Origin',(74.,19.,-31.1547005383792));
#8043=CARTESIAN_POINT('',(72.,3.,-32.3094010767585));
#8044=CARTESIAN_POINT('',(74.,3.,-31.1547005383792));
#8045=CARTESIAN_POINT('',(72.,19.,-32.3094010767585));
#8046=CARTESIAN_POINT('',(72.,19.,-32.3094010767585));
#8047=CARTESIAN_POINT('',(74.,19.,-31.1547005383792));
#8048=CARTESIAN_POINT('Origin',(72.,19.,-32.3094010767585));
#8049=CARTESIAN_POINT('',(70.0000000000001,3.,-31.1547005383792));
#8050=CARTESIAN_POINT('',(72.,3.,-32.3094010767585));
#8051=CARTESIAN_POINT('',(70.0000000000001,19.,-31.1547005383792));
#8052=CARTESIAN_POINT('',(70.0000000000001,19.,-31.1547005383792));
#8053=CARTESIAN_POINT('',(72.,19.,-32.3094010767585));
#8054=CARTESIAN_POINT('Origin',(70.0000000000001,19.,-31.1547005383792));
#8055=CARTESIAN_POINT('',(70.0000000000001,3.,-28.8452994616208));
#8056=CARTESIAN_POINT('',(70.0000000000001,3.,-31.1547005383792));
#8057=CARTESIAN_POINT('',(70.0000000000001,19.,-28.8452994616208));
#8058=CARTESIAN_POINT('',(70.0000000000001,19.,-28.8452994616208));
#8059=CARTESIAN_POINT('',(70.0000000000001,19.,-31.1547005383792));
#8060=CARTESIAN_POINT('Origin',(70.0000000000001,19.,-28.8452994616208));
#8061=CARTESIAN_POINT('',(70.0000000000001,3.,-28.8452994616208));
#8062=CARTESIAN_POINT('',(70.0000000000001,19.,-28.8452994616208));
#8063=CARTESIAN_POINT('Origin',(74.,19.,-28.8452994616208));
#8064=CARTESIAN_POINT('Origin',(74.,3.,-28.8452994616208));
#12948=UNCERTAINTY_MEASURE_WITH_UNIT(LENGTH_MEASURE(0.01),#12967,
'DISTANCE_ACCURACY_VALUE',
'Maximum model space distance between geometric entities at asserted c
onnectivities');
#12956=UNCERTAINTY_MEASURE_WITH_UNIT(LENGTH_MEASURE(0.01),#12967,
'DISTANCE_ACCURACY_VALUE',
'Maximum model space distance between geometric entities at asserted c
onnectivities');
#12958=(
GEOMETRIC_REPRESENTATION_CONTEXT(3)
GLOBAL_UNCERTAINTY_ASSIGNED_CONTEXT((#12948))
GLOBAL_UNIT_ASSIGNED_CONTEXT((#12967,#12969,#12970))
REPRESENTATION_CONTEXT('','3D')
);
#12966=(
GEOMETRIC_REPRESENTATION_CONTEXT(3)
GLOBAL_UNCERTAINTY_ASSIGNED_CONTEXT((#12956))
GLOBAL_UNIT_ASSIGNED_CONTEXT((#12967,#12969,#12970))
REPRESENTATION_CONTEXT('','3D')
);
#12967=(
LENGTH_UNIT()
NAMED_UNIT(*)
SI_UNIT(.MILLI.,.METRE.)
);
#12969=(
NAMED_UNIT(*)
PLANE_ANGLE_UNIT()
SI_UNIT($,.RADIAN.)
);
#12970=(
NAMED_UNIT(*)
SI_UNIT($,.STERADIAN.)
SOLID_ANGLE_UNIT()
);
#12972=SHAPE_DEFINITION_REPRESENTATION(#12981,#13025);
#12981=PRODUCT_DEFINITION_SHAPE('',$,#13035);
#13025=SHAPE_REPRESENTATION('',(#5680),#12958);
#13033=PRODUCT_DEFINITION_CONTEXT('part definition',#13062,'design');
#13035=PRODUCT_DEFINITION('Base Frame','Base Frame',#13044,#13033);
#13044=PRODUCT_DEFINITION_FORMATION('',$,#13065);
#13062=APPLICATION_CONTEXT(
'Core Data for Automotive Mechanical Design Process');
#13063=PRODUCT_CONTEXT('part definition',#13062,'mechanical');
#13065=PRODUCT('Base Frame','Base Frame',$,(#13063));
#13074=PRESENTATION_STYLE_ASSIGNMENT((#13079));
#13079=SURFACE_STYLE_USAGE(.BOTH.,#13084);
#13084=SURFACE_SIDE_STYLE('',(#13089));
#13089=SURFACE_STYLE_FILL_AREA(#13094);
#13094=FILL_AREA_STYLE('Opaque(20,51,87)',(#13099));
#13099=FILL_AREA_STYLE_COLOUR('Opaque(20,51,87)',#13104);
#13104=COLOUR_RGB('Opaque(20,51,87)',0.0784313725490196,0.2,0.341176470588235);
ENDSEC;
END-ISO-10303-21;
